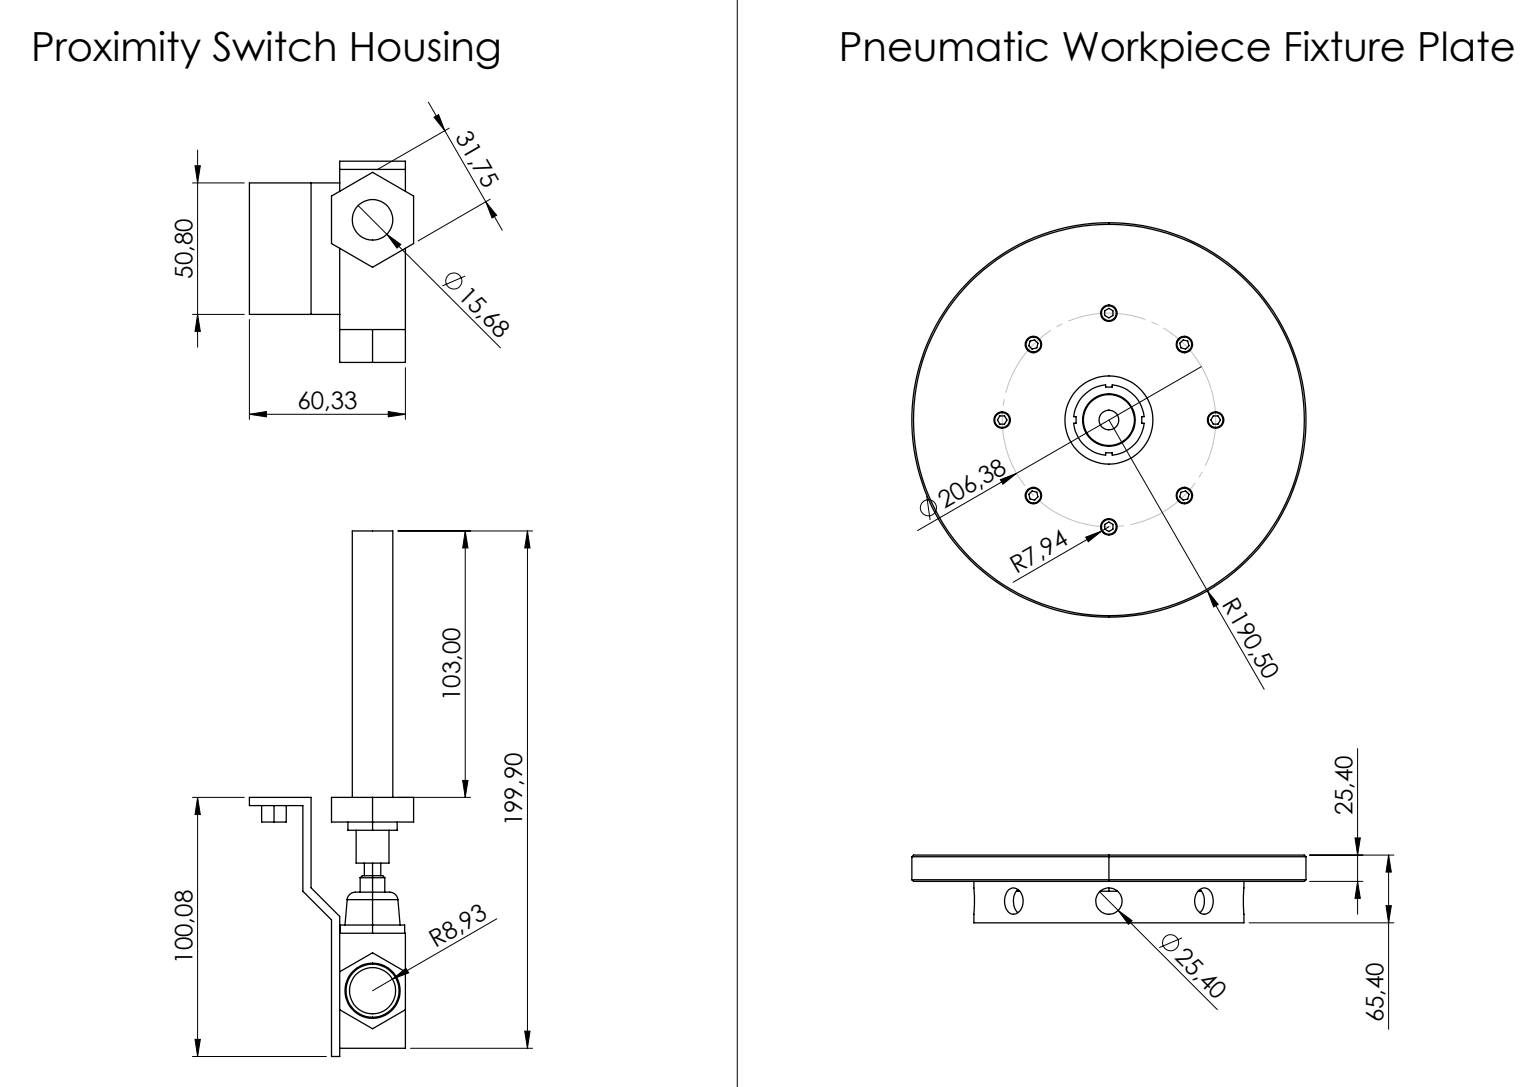
ISO-10303-21;
HEADER;
FILE_DESCRIPTION (('STEP AP214'),
    '1' );
FILE_NAME ('Proximity Switch Housing.step',
    '2026-10-07T11:37:37',
    ( '' ),
    ( '' ),
    'SwSTEP 2.0',
    'SolidWorks 2020',
    '' );
FILE_SCHEMA (( 'AUTOMOTIVE_DESIGN' ));
ENDSEC;

DATA;
#12=AXIS2_PLACEMENT_3D ( 'NONE', #30544, #63723, #30982 ) ;
#15=EDGE_LOOP ( 'NONE', ( #73624, #35100, #2042, #65680 ) ) ;
#24=CARTESIAN_POINT ( 'NONE',  ( 199.3900000000000148, 46.38749999999999574, -50.79999999999999716 ) ) ;
#109=ORIENTED_EDGE ( 'NONE', *, *, #12463, .F. ) ;
#113=DIRECTION ( 'NONE',  ( -1.000000000000000000, 0.000000000000000000, 0.000000000000000000 ) ) ;
#254=EDGE_CURVE ( 'NONE', #38623, #81994, #26176, .T. ) ;
#275=AXIS2_PLACEMENT_3D ( 'NONE', #19482, #13126, #74898 ) ;
#303=EDGE_CURVE ( 'NONE', #54782, #72244, #41574, .T. ) ;
#324=CARTESIAN_POINT ( 'NONE',  ( 199.3900000000000148, 59.08750000000000568, -50.79999999999999716 ) ) ;
#330=VECTOR ( 'NONE', #57470, 1000.000000000000000 ) ;
#479=LINE ( 'NONE', #75450, #54659 ) ;
#499=AXIS2_PLACEMENT_3D ( 'NONE', #66233, #38984, #31726 ) ;
#526=LINE ( 'NONE', #77290, #28220 ) ;
#540=DIRECTION ( 'NONE',  ( -1.000000000000000000, 0.000000000000000000, 0.000000000000000000 ) ) ;
#574=ORIENTED_EDGE ( 'NONE', *, *, #33050, .F. ) ;
#662=VECTOR ( 'NONE', #54108, 1000.000000000000000 ) ;
#687=VECTOR ( 'NONE', #72878, 1000.000000000000000 ) ;
#739=EDGE_CURVE ( 'NONE', #86672, #54266, #21377, .T. ) ;
#780=DIRECTION ( 'NONE',  ( -1.000000000000000000, 0.000000000000000000, 0.000000000000000000 ) ) ;
#832=PLANE ( 'NONE',  #52859 ) ;
#845=ORIENTED_EDGE ( 'NONE', *, *, #49423, .F. ) ;
#869=ADVANCED_FACE ( 'NONE', ( #70025 ), #14620, .F. ) ;
#917=DIRECTION ( 'NONE',  ( -1.000000000000000000, 3.651563665954184899E-16, 0.000000000000000000 ) ) ;
#1006=EDGE_CURVE ( 'NONE', #6675, #59868, #43643, .T. ) ;
#1029=EDGE_CURVE ( 'NONE', #69678, #54710, #73477, .T. ) ;
#1074=AXIS2_PLACEMENT_3D ( 'NONE', #83789, #85142, #1565 ) ;
#1102=EDGE_LOOP ( 'NONE', ( #66047, #88508, #70924, #49259 ) ) ;
#1110=CYLINDRICAL_SURFACE ( 'NONE', #1074, 3.174999999999997158 ) ;
#1150=ORIENTED_EDGE ( 'NONE', *, *, #9525, .F. ) ;
#1247=CIRCLE ( 'NONE', #51976, 6.647542495715439870 ) ;
#1266=CIRCLE ( 'NONE', #37574, 4.762500000000002842 ) ;
#1356=FACE_BOUND ( 'NONE', #25770, .T. ) ;
#1386=EDGE_CURVE ( 'NONE', #86177, #20936, #44319, .T. ) ;
#1433=CARTESIAN_POINT ( 'NONE',  ( 270.8910000000000196, 40.03750000000000142, -2.032000000000000028 ) ) ;
#1445=CARTESIAN_POINT ( 'NONE',  ( 183.5150000000000148, 36.86249999999999716, -53.61543552338530105 ) ) ;
#1493=EDGE_CURVE ( 'NONE', #9584, #8177, #75540, .T. ) ;
#1565=DIRECTION ( 'NONE',  ( 0.000000000000000000, 0.000000000000000000, 1.000000000000000000 ) ) ;
#1642=AXIS2_PLACEMENT_3D ( 'NONE', #6574, #49231, #61972 ) ;
#1645=PLANE ( 'NONE',  #8923 ) ;
#1649=LINE ( 'NONE', #29349, #83719 ) ;
#1671=ORIENTED_EDGE ( 'NONE', *, *, #58217, .F. ) ;
#1703=ORIENTED_EDGE ( 'NONE', *, *, #9525, .T. ) ;
#1756=ORIENTED_EDGE ( 'NONE', *, *, #68896, .F. ) ;
#1859=EDGE_LOOP ( 'NONE', ( #80684, #22830, #9417, #17174 ) ) ;
#1868=CARTESIAN_POINT ( 'NONE',  ( 219.9639999999999986, 40.03750000000000142, -58.73749999999999716 ) ) ;
#1873=VECTOR ( 'NONE', #29964, 1000.000000000000000 ) ;
#1909=LINE ( 'NONE', #56399, #17152 ) ;
#2007=DIRECTION ( 'NONE',  ( 1.000000000000000000, 0.000000000000000000, 0.000000000000000000 ) ) ;
#2029=ORIENTED_EDGE ( 'NONE', *, *, #65942, .T. ) ;
#2031=ORIENTED_EDGE ( 'NONE', *, *, #43091, .T. ) ;
#2042=ORIENTED_EDGE ( 'NONE', *, *, #74462, .F. ) ;
#2067=DIRECTION ( 'NONE',  ( 1.000000000000000000, 0.000000000000000000, 0.000000000000000000 ) ) ;
#2111=DIRECTION ( 'NONE',  ( -1.000000000000000000, 0.000000000000000000, -2.108231265501709878E-16 ) ) ;
#2112=AXIS2_PLACEMENT_3D ( 'NONE', #54801, #19863, #47549 ) ;
#2145=STYLED_ITEM ( 'NONE', ( #66142 ), #80104 ) ;
#2148=VECTOR ( 'NONE', #84868, 1000.000000000000000 ) ;
#2157=DIRECTION ( 'NONE',  ( -7.136255983449500255E-16, 0.000000000000000000, -1.000000000000000000 ) ) ;
#2234=ADVANCED_FACE ( 'NONE', ( #77753 ), #41852, .T. ) ;
#2261=LINE ( 'NONE', #50383, #1873 ) ;
#2282=CARTESIAN_POINT ( 'NONE',  ( 177.1649999999999920, 5.112500000000000711, -58.73749999999999716 ) ) ;
#2363=VECTOR ( 'NONE', #69256, 1000.000000000000000 ) ;
#2380=VECTOR ( 'NONE', #46487, 1000.000000000000000 ) ;
#2407=CARTESIAN_POINT ( 'NONE',  ( 270.8910000000000196, 40.03750000000000142, -67.11950000000000216 ) ) ;
#2427=AXIS2_PLACEMENT_3D ( 'NONE', #81072, #79730, #72455 ) ;
#2428=AXIS2_PLACEMENT_3D ( 'NONE', #75182, #5245, #32934 ) ;
#2439=DIRECTION ( 'NONE',  ( 1.000000000000000000, 0.000000000000000000, 0.000000000000000000 ) ) ;
#2482=CARTESIAN_POINT ( 'NONE',  ( 204.2160000000000082, 52.73749999999999716, -40.48124999999945572 ) ) ;
#2499=EDGE_CURVE ( 'NONE', #28622, #16389, #84475, .T. ) ;
#2686=DIRECTION ( 'NONE',  ( 0.000000000000000000, 0.000000000000000000, 1.000000000000000000 ) ) ;
#2696=LINE ( 'NONE', #16767, #70704 ) ;
#2727=VERTEX_POINT ( 'NONE', #73946 ) ;
#2742=DIRECTION ( 'NONE',  ( 0.000000000000000000, 0.000000000000000000, -1.000000000000000000 ) ) ;
#2848=CARTESIAN_POINT ( 'NONE',  ( 226.4410000000000025, 40.03750000000000142, 10.66800000000000104 ) ) ;
#2953=VERTEX_POINT ( 'NONE', #86482 ) ;
#2982=VERTEX_POINT ( 'NONE', #59630 ) ;
#2985=VERTEX_POINT ( 'NONE', #38308 ) ;
#3007=AXIS2_PLACEMENT_3D ( 'NONE', #78593, #71762, #83602 ) ;
#3067=DIRECTION ( 'NONE',  ( -1.000000000000000000, 0.000000000000000000, -2.108231265501709878E-16 ) ) ;
#3078=VECTOR ( 'NONE', #53283, 1000.000000000000000 ) ;
#3128=ORIENTED_EDGE ( 'NONE', *, *, #41850, .T. ) ;
#3145=DIRECTION ( 'NONE',  ( 0.000000000000000000, -0.8660254037844383745, -0.5000000000000003331 ) ) ;
#3249=VECTOR ( 'NONE', #48898, 1000.000000000000000 ) ;
#3299=SURFACE_STYLE_USAGE ( .BOTH. , #17812 ) ;
#3320=ORIENTED_EDGE ( 'NONE', *, *, #23264, .T. ) ;
#3451=CARTESIAN_POINT ( 'NONE',  ( 223.2659999999999911, 52.73749999999999716, -32.00399999999999778 ) ) ;
#3471=EDGE_CURVE ( 'NONE', #54390, #10350, #12838, .T. ) ;
#3643=CARTESIAN_POINT ( 'NONE',  ( 177.1649999999999920, 5.112500000000000711, -7.937500000000000000 ) ) ;
#3651=CIRCLE ( 'NONE', #41367, 10.26166025953212468 ) ;
#3667=CARTESIAN_POINT ( 'NONE',  ( 223.2659999999999911, 52.73749999999999716, -44.45000000000000284 ) ) ;
#3711=DIRECTION ( 'NONE',  ( 1.000000000000000000, 0.000000000000000000, 0.000000000000000000 ) ) ;
#3736=( LENGTH_UNIT ( ) NAMED_UNIT ( * ) SI_UNIT ( .MILLI., .METRE. ) );
#3760=ORIENTED_EDGE ( 'NONE', *, *, #23279, .T. ) ;
#3831=VERTEX_POINT ( 'NONE', #85830 ) ;
#3838=VECTOR ( 'NONE', #48336, 1000.000000000000000 ) ;
#3867=CARTESIAN_POINT ( 'NONE',  ( 173.9899999999999807, 52.73749999999999716, -52.28750000000000142 ) ) ;
#3937=ORIENTED_EDGE ( 'NONE', *, *, #41802, .T. ) ;
#4117=CARTESIAN_POINT ( 'NONE',  ( 173.9900000000000091, 52.73749999999999716, -62.78087104677060637 ) ) ;
#4160=CARTESIAN_POINT ( 'NONE',  ( 223.2659999999999911, 52.73749999999999716, -32.00399999999999778 ) ) ;
#4201=CARTESIAN_POINT ( 'NONE',  ( 177.1649999999999920, 14.63749999999999929, -52.38749999999999574 ) ) ;
#4243=DIRECTION ( 'NONE',  ( 1.000000000000000000, -0.000000000000000000, 2.108231265501710124E-16 ) ) ;
#4288=CARTESIAN_POINT ( 'NONE',  ( 183.5150000000000148, 52.73749999999999716, -26.11912895322935313 ) ) ;
#4323=ORIENTED_EDGE ( 'NONE', *, *, #74462, .T. ) ;
#4489=EDGE_CURVE ( 'NONE', #56634, #71751, #79798, .T. ) ;
#4515=ORIENTED_EDGE ( 'NONE', *, *, #27620, .F. ) ;
#4572=VECTOR ( 'NONE', #22994, 1000.000000000000000 ) ;
#4580=EDGE_LOOP ( 'NONE', ( #33206, #53501, #39020, #4323, #51486, #11776 ) ) ;
#4611=VERTEX_POINT ( 'NONE', #71043 ) ;
#4729=PLANE ( 'NONE',  #67107 ) ;
#4776=EDGE_CURVE ( 'NONE', #88384, #78380, #88690, .T. ) ;
#4790=EDGE_CURVE ( 'NONE', #2982, #52784, #78320, .T. ) ;
#4815=DIRECTION ( 'NONE',  ( -1.000000000000000000, 0.000000000000000000, 0.000000000000000000 ) ) ;
#4819=ORIENTED_EDGE ( 'NONE', *, *, #87208, .F. ) ;
#4821=CIRCLE ( 'NONE', #38214, 4.762500000000002842 ) ;
#4869=VECTOR ( 'NONE', #26634, 1000.000000000000000 ) ;
#4881=DIRECTION ( 'NONE',  ( 0.000000000000000000, 0.000000000000000000, 1.000000000000000000 ) ) ;
#4896=DIRECTION ( 'NONE',  ( -7.980413499659419871E-32, 1.000000000000000000, 3.785359618865284342E-16 ) ) ;
#4921=FACE_OUTER_BOUND ( 'NONE', #41166, .T. ) ;
#4941=EDGE_CURVE ( 'NONE', #64462, #86177, #25609, .T. ) ;
#4972=LINE ( 'NONE', #60365, #32186 ) ;
#5049=LINE ( 'NONE', #45024, #11322 ) ;
#5066=ORIENTED_EDGE ( 'NONE', *, *, #16121, .T. ) ;
#5245=DIRECTION ( 'NONE',  ( 0.000000000000000000, -1.000000000000000000, 0.000000000000000000 ) ) ;
#5445=LINE ( 'NONE', #68114, #10349 ) ;
#5493=DIRECTION ( 'NONE',  ( 0.000000000000000000, 0.000000000000000000, 1.000000000000000000 ) ) ;
#5642=DIRECTION ( 'NONE',  ( 1.000000000000000000, 0.000000000000000000, 0.000000000000000000 ) ) ;
#5664=EDGE_CURVE ( 'NONE', #22107, #30158, #47504, .T. ) ;
#5881=CARTESIAN_POINT ( 'NONE',  ( 173.9900000000000091, 5.112500000000000711, -7.937500000000000000 ) ) ;
#5942=CARTESIAN_POINT ( 'NONE',  ( 223.2659999999999911, 36.86249999999999716, -2.032000000000000028 ) ) ;
#6110=DIRECTION ( 'NONE',  ( -1.000000000000000000, 0.000000000000000000, 0.000000000000000000 ) ) ;
#6112=DIRECTION ( 'NONE',  ( -1.000000000000000000, 0.000000000000000000, 0.000000000000000000 ) ) ;
#6116=ORIENTED_EDGE ( 'NONE', *, *, #76740, .T. ) ;
#6360=VERTEX_POINT ( 'NONE', #29660 ) ;
#6379=EDGE_LOOP ( 'NONE', ( #29242, #79517, #85233, #49817, #49646, #1703 ) ) ;
#6410=EDGE_CURVE ( 'NONE', #78558, #73485, #7548, .T. ) ;
#6437=VECTOR ( 'NONE', #780, 1000.000000000000000 ) ;
#6476=AXIS2_PLACEMENT_3D ( 'NONE', #8190, #42680, #69522 ) ;
#6480=CIRCLE ( 'NONE', #74626, 12.44599999999999795 ) ;
#6490=DIRECTION ( 'NONE',  ( -0.8660254037844387076, 0.4999999999999998890, 0.000000000000000000 ) ) ;
#6491=EDGE_CURVE ( 'NONE', #47477, #14995, #80961, .T. ) ;
#6512=DIRECTION ( 'NONE',  ( 0.000000000000000000, 0.000000000000000000, -1.000000000000000000 ) ) ;
#6526=CIRCLE ( 'NONE', #45655, 3.174999999999997158 ) ;
#6546=LINE ( 'NONE', #81085, #16069 ) ;
#6574=CARTESIAN_POINT ( 'NONE',  ( 183.5150000000000148, 14.63749999999999929, -14.28749999999999964 ) ) ;
#6654=DIRECTION ( 'NONE',  ( 0.7071067811865504593, 0.000000000000000000, 0.7071067811865445751 ) ) ;
#6662=VECTOR ( 'NONE', #57712, 1000.000000000000000 ) ;
#6671=DIRECTION ( 'NONE',  ( 0.000000000000000000, 0.000000000000000000, -1.000000000000000000 ) ) ;
#6675=VERTEX_POINT ( 'NONE', #55889 ) ;
#6744=CARTESIAN_POINT ( 'NONE',  ( 183.5150000000000148, 68.61249999999999716, -35.28456447661459805 ) ) ;
#6795=EDGE_CURVE ( 'NONE', #65795, #61431, #32119, .T. ) ;
#6839=VECTOR ( 'NONE', #25383, 1000.000000000000000 ) ;
#6841=ORIENTED_EDGE ( 'NONE', *, *, #55333, .F. ) ;
#6894=LINE ( 'NONE', #22330, #26794 ) ;
#7063=ORIENTED_EDGE ( 'NONE', *, *, #81554, .T. ) ;
#7112=DIRECTION ( 'NONE',  ( 0.000000000000000000, 0.000000000000000000, 1.000000000000000000 ) ) ;
#7131=EDGE_CURVE ( 'NONE', #15176, #54672, #85227, .T. ) ;
#7165=( GEOMETRIC_REPRESENTATION_CONTEXT ( 3 ) GLOBAL_UNCERTAINTY_ASSIGNED_CONTEXT ( ( #28762 ) ) GLOBAL_UNIT_ASSIGNED_CONTEXT ( ( #3736, #71897, #44158 ) ) REPRESENTATION_CONTEXT ( 'NONE', 'WORKASPACE' ) );
#7203=ORIENTED_EDGE ( 'NONE', *, *, #5664, .F. ) ;
#7223=ORIENTED_EDGE ( 'NONE', *, *, #30920, .T. ) ;
#7285=ORIENTED_EDGE ( 'NONE', *, *, #44170, .T. ) ;
#7290=FACE_OUTER_BOUND ( 'NONE', #87103, .T. ) ;
#7453=ORIENTED_EDGE ( 'NONE', *, *, #30720, .T. ) ;
#7485=EDGE_CURVE ( 'NONE', #81994, #84665, #6546, .T. ) ;
#7493=LINE ( 'NONE', #35178, #50384 ) ;
#7548=CIRCLE ( 'NONE', #19148, 9.810460662156732070 ) ;
#7583=CARTESIAN_POINT ( 'NONE',  ( 204.2160000000000082, 52.73749999999999716, -40.48124999999945572 ) ) ;
#7617=ORIENTED_EDGE ( 'NONE', *, *, #1493, .F. ) ;
#7626=DIRECTION ( 'NONE',  ( 0.000000000000000000, 0.000000000000000000, 1.000000000000000000 ) ) ;
#7653=CARTESIAN_POINT ( 'NONE',  ( 270.8910000000000196, 65.43750000000000000, -2.032000000000000028 ) ) ;
#7681=PLANE ( 'NONE',  #27434 ) ;
#7809=FACE_OUTER_BOUND ( 'NONE', #85300, .T. ) ;
#7840=DIRECTION ( 'NONE',  ( 0.000000000000000000, 0.000000000000000000, -1.000000000000000000 ) ) ;
#7843=DIRECTION ( 'NONE',  ( 0.000000000000000000, 0.000000000000000000, 1.000000000000000000 ) ) ;
#7994=PLANE ( 'NONE',  #50960 ) ;
#8009=AXIS2_PLACEMENT_3D ( 'NONE', #64340, #2111, #29821 ) ;
#8064=EDGE_LOOP ( 'NONE', ( #83886, #3320, #1150, #32681, #73638, #52637, #41775, #28996 ) ) ;
#8075=DIRECTION ( 'NONE',  ( -1.000000000000000000, 0.000000000000000000, -2.108231265501709878E-16 ) ) ;
#8113=ORIENTED_EDGE ( 'NONE', *, *, #80354, .F. ) ;
#8158=EDGE_LOOP ( 'NONE', ( #20110, #78432, #2029, #49660 ) ) ;
#8177=VERTEX_POINT ( 'NONE', #79977 ) ;
#8190=CARTESIAN_POINT ( 'NONE',  ( 183.5150000000000148, 14.63749999999999929, -52.38749999999999574 ) ) ;
#8302=FACE_BOUND ( 'NONE', #23000, .T. ) ;
#8349=EDGE_CURVE ( 'NONE', #47225, #2985, #5445, .T. ) ;
#8374=ADVANCED_FACE ( 'NONE', ( #46298, #31794, #12251 ), #39944, .F. ) ;
#8429=ORIENTED_EDGE ( 'NONE', *, *, #4489, .F. ) ;
#8455=CARTESIAN_POINT ( 'NONE',  ( 248.6659999999999968, 52.73749999999999716, 10.66800000000000104 ) ) ;
#8461=ORIENTED_EDGE ( 'NONE', *, *, #57159, .T. ) ;
#8474=DIRECTION ( 'NONE',  ( -1.000000000000000000, 0.000000000000000000, 5.463695987328529395E-16 ) ) ;
#8565=VERTEX_POINT ( 'NONE', #56243 ) ;
#8726=CARTESIAN_POINT ( 'NONE',  ( 270.8910000000000196, 40.03750000000000142, -7.937500000000000000 ) ) ;
#8761=PLANE ( 'NONE',  #54111 ) ;
#8850=DIRECTION ( 'NONE',  ( 0.000000000000000000, 0.000000000000000000, 1.000000000000000000 ) ) ;
#8864=CARTESIAN_POINT ( 'NONE',  ( 205.0097499999990305, 52.73749999999999716, -49.21249999999999858 ) ) ;
#8923=AXIS2_PLACEMENT_3D ( 'NONE', #50209, #28430, #36611 ) ;
#8938=ORIENTED_EDGE ( 'NONE', *, *, #10937, .F. ) ;
#9003=ORIENTED_EDGE ( 'NONE', *, *, #13599, .F. ) ;
#9037=VERTEX_POINT ( 'NONE', #60159 ) ;
#9061=ORIENTED_EDGE ( 'NONE', *, *, #13025, .T. ) ;
#9154=VECTOR ( 'NONE', #28074, 1000.000000000000000 ) ;
#9187=CARTESIAN_POINT ( 'NONE',  ( 183.5150000000000148, 14.63749999999999929, -9.525000000000000355 ) ) ;
#9237=CARTESIAN_POINT ( 'NONE',  ( 263.3306968374159851, 52.73749999999999716, -2.032000000000000028 ) ) ;
#9264=CARTESIAN_POINT ( 'NONE',  ( 205.0097499999990305, 52.73749999999999716, -44.45000000000000284 ) ) ;
#9417=ORIENTED_EDGE ( 'NONE', *, *, #83533, .T. ) ;
#9525=EDGE_CURVE ( 'NONE', #62756, #15555, #526, .T. ) ;
#9570=DIRECTION ( 'NONE',  ( -1.000000000000000000, 0.000000000000000000, -2.108231265501709878E-16 ) ) ;
#9577=LINE ( 'NONE', #87220, #70374 ) ;
#9584=VERTEX_POINT ( 'NONE', #55916 ) ;
#9589=EDGE_CURVE ( 'NONE', #84035, #35999, #6894, .T. ) ;
#9637=ORIENTED_EDGE ( 'NONE', *, *, #10817, .T. ) ;
#9639=DIRECTION ( 'NONE',  ( 0.000000000000000000, -1.000000000000000000, 0.000000000000000000 ) ) ;
#9649=LINE ( 'NONE', #2848, #27057 ) ;
#9678=VECTOR ( 'NONE', #2686, 1000.000000000000000 ) ;
#9707=DIRECTION ( 'NONE',  ( 1.000000000000000000, 0.000000000000000000, 0.000000000000000000 ) ) ;
#9795=CIRCLE ( 'NONE', #75074, 12.44599999999999795 ) ;
#9866=ORIENTED_EDGE ( 'NONE', *, *, #41587, .F. ) ;
#9890=CARTESIAN_POINT ( 'NONE',  ( 257.5940999999999690, 52.73749999999999716, 10.66800000000000104 ) ) ;
#9978=DIRECTION ( 'NONE',  ( 0.000000000000000000, 0.000000000000000000, 1.000000000000000000 ) ) ;
#9984=CARTESIAN_POINT ( 'NONE',  ( 183.5150000000000148, 68.61249999999999716, -53.61543552338530105 ) ) ;
#10068=AXIS2_PLACEMENT_3D ( 'NONE', #58861, #24807, #66576 ) ;
#10192=ORIENTED_EDGE ( 'NONE', *, *, #9589, .F. ) ;
#10279=ORIENTED_EDGE ( 'NONE', *, *, #62430, .T. ) ;
#10290=ORIENTED_EDGE ( 'NONE', *, *, #57784, .T. ) ;
#10349=VECTOR ( 'NONE', #13155, 1000.000000000000000 ) ;
#10350=VERTEX_POINT ( 'NONE', #3451 ) ;
#10356=DIRECTION ( 'NONE',  ( 2.108231265501709878E-16, 0.000000000000000000, -1.000000000000000000 ) ) ;
#10368=DIRECTION ( 'NONE',  ( 0.000000000000000000, 0.000000000000000000, 1.000000000000000000 ) ) ;
#10440=DIRECTION ( 'NONE',  ( 0.000000000000000000, 0.000000000000000000, 1.000000000000000000 ) ) ;
#10536=CIRCLE ( 'NONE', #22159, 4.762500000000002842 ) ;
#10560=CARTESIAN_POINT ( 'NONE',  ( 186.6899999999999977, 59.08750000000000568, -50.79999999999999716 ) ) ;
#10635=ADVANCED_FACE ( 'NONE', ( #78327 ), #1110, .T. ) ;
#10645=CARTESIAN_POINT ( 'NONE',  ( 204.2160000000000082, 52.73749999999999716, -44.45000000000000284 ) ) ;
#10666=DIRECTION ( 'NONE',  ( 0.000000000000000000, 1.000000000000000000, 5.463695987328529395E-16 ) ) ;
#10732=( NAMED_UNIT ( * ) PLANE_ANGLE_UNIT ( ) SI_UNIT ( $, .RADIAN. ) );
#10739=LINE ( 'NONE', #23516, #49588 ) ;
#10781=AXIS2_PLACEMENT_3D ( 'NONE', #85648, #66056, #17039 ) ;
#10817=EDGE_CURVE ( 'NONE', #2727, #42703, #82392, .T. ) ;
#10845=VERTEX_POINT ( 'NONE', #82343 ) ;
#10919=EDGE_CURVE ( 'NONE', #32855, #84272, #82794, .T. ) ;
#10937=EDGE_CURVE ( 'NONE', #25134, #76956, #36857, .T. ) ;
#10944=DIRECTION ( 'NONE',  ( 1.000000000000000000, 0.000000000000000000, -5.463695987328529395E-16 ) ) ;
#10984=CIRCLE ( 'NONE', #21120, 9.524999999999998579 ) ;
#10990=( NAMED_UNIT ( * ) PLANE_ANGLE_UNIT ( ) SI_UNIT ( $, .RADIAN. ) );
#11060=FACE_OUTER_BOUND ( 'NONE', #54415, .T. ) ;
#11080=DIRECTION ( 'NONE',  ( 0.9961946980917455452, 0.000000000000000000, 0.08715574274765836016 ) ) ;
#11094=DIRECTION ( 'NONE',  ( 0.000000000000000000, 0.000000000000000000, 1.000000000000000000 ) ) ;
#11154=CARTESIAN_POINT ( 'NONE',  ( 241.3336515812914911, 65.43750000000000000, -2.032000000000000028 ) ) ;
#11195=VERTEX_POINT ( 'NONE', #4117 ) ;
#11229=VECTOR ( 'NONE', #22249, 1000.000000000000000 ) ;
#11246=ORIENTED_EDGE ( 'NONE', *, *, #42075, .F. ) ;
#11253=PLANE ( 'NONE',  #83559 ) ;
#11306=VECTOR ( 'NONE', #80656, 1000.000000000000000 ) ;
#11322=VECTOR ( 'NONE', #18675, 1000.000000000000000 ) ;
#11404=ORIENTED_EDGE ( 'NONE', *, *, #32887, .F. ) ;
#11437=EDGE_CURVE ( 'NONE', #30447, #18949, #70377, .T. ) ;
#11451=DIRECTION ( 'NONE',  ( -1.825781832977099352E-16, 0.4999999999999998890, 0.8660254037844387076 ) ) ;
#11465=CARTESIAN_POINT ( 'NONE',  ( 199.3900000000000148, 52.73749999999999716, -44.45000000000000284 ) ) ;
#11513=LINE ( 'NONE', #39209, #44408 ) ;
#11535=EDGE_CURVE ( 'NONE', #74351, #54417, #57629, .T. ) ;
#11587=AXIS2_PLACEMENT_3D ( 'NONE', #32865, #46926, #31972 ) ;
#11687=DIRECTION ( 'NONE',  ( -2.108231265501709878E-16, 5.463695987328529395E-16, 1.000000000000000000 ) ) ;
#11776=ORIENTED_EDGE ( 'NONE', *, *, #45978, .T. ) ;
#11779=ORIENTED_EDGE ( 'NONE', *, *, #64075, .T. ) ;
#11829=ADVANCED_FACE ( 'NONE', ( #40311 ), #27257, .T. ) ;
#11853=AXIS2_PLACEMENT_3D ( 'NONE', #81263, #79476, #31288 ) ;
#11871=CARTESIAN_POINT ( 'NONE',  ( 204.2160000000000082, 52.73749999999999716, -48.41875000000000284 ) ) ;
#11875=AXIS2_PLACEMENT_3D ( 'NONE', #17373, #86429, #45056 ) ;
#11891=EDGE_CURVE ( 'NONE', #52784, #11922, #48008, .T. ) ;
#11894=FACE_OUTER_BOUND ( 'NONE', #30527, .T. ) ;
#11922=VERTEX_POINT ( 'NONE', #41200 ) ;
#11931=CARTESIAN_POINT ( 'NONE',  ( 173.9900000000000091, 52.73749999999999716, -26.11912895322935313 ) ) ;
#11948=DIRECTION ( 'NONE',  ( 1.000000000000000000, 1.314511288311335947E-16, 0.000000000000000000 ) ) ;
#11981=ORIENTED_EDGE ( 'NONE', *, *, #17799, .T. ) ;
#12025=DIRECTION ( 'NONE',  ( 0.000000000000000000, 0.000000000000000000, -1.000000000000000000 ) ) ;
#12026=CARTESIAN_POINT ( 'NONE',  ( 183.5150000000000148, 14.63749999999999929, -52.38749999999999574 ) ) ;
#12175=EDGE_CURVE ( 'NONE', #83823, #14890, #27368, .T. ) ;
#12249=LINE ( 'NONE', #61282, #13166 ) ;
#12251=FACE_BOUND ( 'NONE', #56681, .T. ) ;
#12273=DIRECTION ( 'NONE',  ( 0.000000000000000000, -0.8660254037844383745, -0.5000000000000003331 ) ) ;
#12325=EDGE_CURVE ( 'NONE', #83557, #61431, #35513, .T. ) ;
#12329=PLANE ( 'NONE',  #33594 ) ;
#12369=CARTESIAN_POINT ( 'NONE',  ( 183.5150000000000148, 52.73749999999999716, -34.92499999999999716 ) ) ;
#12402=VECTOR ( 'NONE', #59601, 1000.000000000000000 ) ;
#12416=CARTESIAN_POINT ( 'NONE',  ( 204.2160000000000082, 52.73749999999999716, -48.41875000000000284 ) ) ;
#12435=CARTESIAN_POINT ( 'NONE',  ( 183.5150000000000148, 68.61249999999999716, -71.94630657015589748 ) ) ;
#12459=ADVANCED_FACE ( 'NONE', ( #85939 ), #87702, .F. ) ;
#12463=EDGE_CURVE ( 'NONE', #17992, #69275, #53138, .T. ) ;
#12464=CARTESIAN_POINT ( 'NONE',  ( 204.2160000000000082, 52.73749999999999716, -39.68750000000000000 ) ) ;
#12470=FACE_OUTER_BOUND ( 'NONE', #60850, .T. ) ;
#12473=EDGE_CURVE ( 'NONE', #66028, #64424, #52875, .T. ) ;
#12496=ORIENTED_EDGE ( 'NONE', *, *, #68896, .T. ) ;
#12522=EDGE_LOOP ( 'NONE', ( #37000, #71430, #23849, #81883 ) ) ;
#12595=ADVANCED_FACE ( 'NONE', ( #40440 ), #68609, .T. ) ;
#12709=DIRECTION ( 'NONE',  ( -1.000000000000000000, 0.000000000000000000, 0.000000000000000000 ) ) ;
#12759=VERTEX_POINT ( 'NONE', #47540 ) ;
#12838=CIRCLE ( 'NONE', #56310, 12.44599999999999795 ) ;
#12839=VERTEX_POINT ( 'NONE', #70244 ) ;
#12943=FACE_BOUND ( 'NONE', #47307, .T. ) ;
#13000=EDGE_CURVE ( 'NONE', #9037, #88384, #15292, .T. ) ;
#13006=CARTESIAN_POINT ( 'NONE',  ( 208.9149999999999920, 28.98850000000000193, -58.73749999999999716 ) ) ;
#13025=EDGE_CURVE ( 'NONE', #54266, #86672, #3651, .T. ) ;
#13087=PLANE ( 'NONE',  #39711 ) ;
#13126=DIRECTION ( 'NONE',  ( 1.000000000000000000, -0.000000000000000000, 2.108231265501710124E-16 ) ) ;
#13142=EDGE_LOOP ( 'NONE', ( #76348, #845, #5066, #62903 ) ) ;
#13155=DIRECTION ( 'NONE',  ( -1.000000000000000000, 0.000000000000000000, -2.108231265501709878E-16 ) ) ;
#13166=VECTOR ( 'NONE', #39942, 1000.000000000000114 ) ;
#13179=AXIS2_PLACEMENT_3D ( 'NONE', #13990, #8075, #7626 ) ;
#13209=CARTESIAN_POINT ( 'NONE',  ( 242.3160000000000025, 65.43750000000000000, -63.94449999999999790 ) ) ;
#13223=VERTEX_POINT ( 'NONE', #11931 ) ;
#13285=ADVANCED_FACE ( 'NONE', ( #80530 ), #45521, .F. ) ;
#13321=ORIENTED_EDGE ( 'NONE', *, *, #49065, .F. ) ;
#13322=LINE ( 'NONE', #62353, #32835 ) ;
#13353=DIRECTION ( 'NONE',  ( 0.4999999999999998890, -0.8660254037844387076, 0.000000000000000000 ) ) ;
#13416=EDGE_LOOP ( 'NONE', ( #1671, #34448, #3937, #43491 ) ) ;
#13430=DIRECTION ( 'NONE',  ( 1.000000000000000000, 0.000000000000000000, 0.000000000000000000 ) ) ;
#13492=ORIENTED_EDGE ( 'NONE', *, *, #31313, .F. ) ;
#13566=VERTEX_POINT ( 'NONE', #1445 ) ;
#13599=EDGE_CURVE ( 'NONE', #24899, #81994, #72714, .T. ) ;
#13682=ADVANCED_FACE ( 'NONE', ( #80424 ), #66776, .T. ) ;
#13802=ADVANCED_FACE ( 'NONE', ( #26344 ), #54013, .F. ) ;
#13830=ORIENTED_EDGE ( 'NONE', *, *, #58217, .T. ) ;
#13905=LINE ( 'NONE', #29336, #330 ) ;
#13920=PLANE ( 'NONE',  #60482 ) ;
#13990=CARTESIAN_POINT ( 'NONE',  ( 173.9899999999999807, 52.73749999999999716, -44.45000000000000284 ) ) ;
#14024=LINE ( 'NONE', #5881, #16272 ) ;
#14146=PLANE ( 'NONE',  #42882 ) ;
#14163=DIRECTION ( 'NONE',  ( -1.000000000000000000, 0.000000000000000000, -2.108231265501709878E-16 ) ) ;
#14191=DIRECTION ( 'NONE',  ( 0.000000000000000000, 0.000000000000000000, 1.000000000000000000 ) ) ;
#14206=EDGE_CURVE ( 'NONE', #40315, #14995, #55588, .T. ) ;
#14228=FACE_OUTER_BOUND ( 'NONE', #85742, .T. ) ;
#14268=VECTOR ( 'NONE', #19301, 1000.000000000000000 ) ;
#14283=FACE_OUTER_BOUND ( 'NONE', #77955, .T. ) ;
#14323=DIRECTION ( 'NONE',  ( 1.000000000000000000, 0.000000000000000000, 0.000000000000000000 ) ) ;
#14335=ORIENTED_EDGE ( 'NONE', *, *, #30920, .F. ) ;
#14351=DIRECTION ( 'NONE',  ( -0.4999999999999998890, -0.8660254037844387076, 0.000000000000000000 ) ) ;
#14364=APPLICATION_CONTEXT ( 'automotive_design' ) ;
#14478=ORIENTED_EDGE ( 'NONE', *, *, #72954, .F. ) ;
#14504=ORIENTED_EDGE ( 'NONE', *, *, #16889, .F. ) ;
#14507=FACE_BOUND ( 'NONE', #88844, .T. ) ;
#14568=AXIS2_PLACEMENT_3D ( 'NONE', #75660, #13430, #24080 ) ;
#14571=ORIENTED_EDGE ( 'NONE', *, *, #19847, .F. ) ;
#14590=CONICAL_SURFACE ( 'NONE', #49373, 10.66799999999999748, 0.08726646259971625186 ) ;
#14620=PLANE ( 'NONE',  #85268 ) ;
#14802=ORIENTED_EDGE ( 'NONE', *, *, #4790, .T. ) ;
#14874=VECTOR ( 'NONE', #11080, 1000.000000000000114 ) ;
#14890=VERTEX_POINT ( 'NONE', #8726 ) ;
#14922=DIRECTION ( 'NONE',  ( 1.000000000000000000, 0.000000000000000000, 2.108231265501709878E-16 ) ) ;
#14938=EDGE_LOOP ( 'NONE', ( #57231, #35001, #27329, #12496 ) ) ;
#14971=CARTESIAN_POINT ( 'NONE',  ( 255.9983484187079910, 40.03750000000000142, -2.032000000000000028 ) ) ;
#14995=VERTEX_POINT ( 'NONE', #81351 ) ;
#15066=CARTESIAN_POINT ( 'NONE',  ( 226.4410000000000025, 52.73749999999999716, -56.89600000000000080 ) ) ;
#15087=DIRECTION ( 'NONE',  ( 1.000000000000000000, 0.000000000000000000, 3.902639990948949304E-17 ) ) ;
#15176=VERTEX_POINT ( 'NONE', #28585 ) ;
#15191=ORIENTED_EDGE ( 'NONE', *, *, #30986, .T. ) ;
#15292=LINE ( 'NONE', #42961, #48617 ) ;
#15302=DIRECTION ( 'NONE',  ( 0.000000000000000000, 0.000000000000000000, 1.000000000000000000 ) ) ;
#15371=CARTESIAN_POINT ( 'NONE',  ( 274.0659999999999741, 40.03750000000000142, -7.937500000000000000 ) ) ;
#15385=CARTESIAN_POINT ( 'NONE',  ( 183.5150000000000148, 52.73749999999999716, -53.97500000000000142 ) ) ;
#15406=VECTOR ( 'NONE', #12273, 1000.000000000000114 ) ;
#15472=LINE ( 'NONE', #2282, #64343 ) ;
#15548=DIRECTION ( 'NONE',  ( 1.000000000000000000, -0.000000000000000000, 2.108231265501710124E-16 ) ) ;
#15549=CLOSED_SHELL ( 'NONE', ( #74468, #26821, #67375, #13285, #28353, #65151, #33795, #77184, #84683, #31319, #24361, #16466, #24022, #52408, #17074, #83080, #48006, #23673, #10635, #83086, #25602, #76205, #35146, #77355, #26934, #26632, #869, #34880, #8374, #85557, #82623, #34634, #56960, #17157, #49843, #28210, #2234, #55795, #57273, #26920, #79966, #49808, #74242, #12595, #63022, #84677, #74077, #32482, #54691, #52567, #12459, #30017, #66107, #13802, #21394, #13682, #16914, #38862, #73046, #31934, #60432, #16702, #81389, #44852, #52770, #28853, #35826, #11829, #34859, #80259, #48452, #23756, #75841, #33007 ) ) ;
#15555=VERTEX_POINT ( 'NONE', #29844 ) ;
#15586=CARTESIAN_POINT ( 'NONE',  ( 70.98999999999998067, 52.73749999999999716, -52.28750000000002274 ) ) ;
#15633=ORIENTED_EDGE ( 'NONE', *, *, #50626, .F. ) ;
#15705=CYLINDRICAL_SURFACE ( 'NONE', #57204, 4.762500000000001066 ) ;
#15816=LINE ( 'NONE', #9890, #2148 ) ;
#15916=FACE_OUTER_BOUND ( 'NONE', #86387, .T. ) ;
#16012=VECTOR ( 'NONE', #80001, 1000.000000000000000 ) ;
#16015=DIRECTION ( 'NONE',  ( 1.000000000000000000, 0.000000000000000000, 0.000000000000000000 ) ) ;
#16040=PRESENTATION_STYLE_ASSIGNMENT (( #3299 ) ) ;
#16069=VECTOR ( 'NONE', #6112, 1000.000000000000000 ) ;
#16111=VECTOR ( 'NONE', #82501, 999.9999999999998863 ) ;
#16121=EDGE_CURVE ( 'NONE', #60085, #4611, #57764, .T. ) ;
#16130=VECTOR ( 'NONE', #18782, 1000.000000000000000 ) ;
#16152=CARTESIAN_POINT ( 'NONE',  ( 226.4410000000000025, 40.03750000000000142, -2.032000000000000028 ) ) ;
#16200=CARTESIAN_POINT ( 'NONE',  ( 223.2659999999999911, 52.73749999999999716, -55.11800000000000210 ) ) ;
#16272=VECTOR ( 'NONE', #75363, 1000.000000000000000 ) ;
#16308=CARTESIAN_POINT ( 'NONE',  ( 177.1649999999999920, 25.81350000000000477, -58.73749999999999716 ) ) ;
#16343=DIRECTION ( 'NONE',  ( 0.000000000000000000, 0.000000000000000000, 1.000000000000000000 ) ) ;
#16361=VECTOR ( 'NONE', #79725, 1000.000000000000000 ) ;
#16373=EDGE_CURVE ( 'NONE', #30447, #6360, #89051, .T. ) ;
#16389=VERTEX_POINT ( 'NONE', #77222 ) ;
#16450=CARTESIAN_POINT ( 'NONE',  ( 183.5150000000000148, 36.86249999999999716, -53.61543552338530105 ) ) ;
#16466=ADVANCED_FACE ( 'NONE', ( #23173 ), #72192, .T. ) ;
#16493=FACE_OUTER_BOUND ( 'NONE', #14938, .T. ) ;
#16518=EDGE_CURVE ( 'NONE', #2985, #13223, #2261, .T. ) ;
#16539=LINE ( 'NONE', #44214, #68538 ) ;
#16552=DIRECTION ( 'NONE',  ( -2.108231265501709878E-16, 0.000000000000000000, 1.000000000000000000 ) ) ;
#16597=DIRECTION ( 'NONE',  ( 0.000000000000000000, 0.000000000000000000, 1.000000000000000000 ) ) ;
#16609=CYLINDRICAL_SURFACE ( 'NONE', #31261, 4.762500000000001066 ) ;
#16683=EDGE_LOOP ( 'NONE', ( #34049, #13492, #37190, #33205 ) ) ;
#16688=CARTESIAN_POINT ( 'NONE',  ( 258.9276602595319901, 52.73749999999999716, -2.903194600000015502 ) ) ;
#16702=ADVANCED_FACE ( 'NONE', ( #33371, #12943 ), #67891, .F. ) ;
#16709=CARTESIAN_POINT ( 'NONE',  ( 242.3160000000000025, 65.43750000000000000, -63.94449999999999790 ) ) ;
#16767=CARTESIAN_POINT ( 'NONE',  ( 210.2301280605339855, 25.81350000000000477, -7.937500000000000000 ) ) ;
#16889=EDGE_CURVE ( 'NONE', #46304, #54672, #49770, .T. ) ;
#16909=VECTOR ( 'NONE', #53092, 1000.000000000000000 ) ;
#16914=ADVANCED_FACE ( 'NONE', ( #14283 ), #41957, .T. ) ;
#16922=DIRECTION ( 'NONE',  ( 0.000000000000000000, 0.000000000000000000, 1.000000000000000000 ) ) ;
#17038=CARTESIAN_POINT ( 'NONE',  ( 183.5150000000000148, 52.73749999999999716, -62.78087104677060637 ) ) ;
#17039=DIRECTION ( 'NONE',  ( 0.000000000000000000, 0.000000000000000000, 1.000000000000000000 ) ) ;
#17074=ADVANCED_FACE ( 'NONE', ( #4921 ), #87155, .T. ) ;
#17082=CARTESIAN_POINT ( 'NONE',  ( 210.5660000000000025, 52.73749999999999716, -44.45000000000000284 ) ) ;
#17091=ORIENTED_EDGE ( 'NONE', *, *, #46147, .F. ) ;
#17152=VECTOR ( 'NONE', #15087, 1000.000000000000000 ) ;
#17157=ADVANCED_FACE ( 'NONE', ( #39872 ), #13087, .F. ) ;
#17174=ORIENTED_EDGE ( 'NONE', *, *, #77090, .F. ) ;
#17179=FACE_OUTER_BOUND ( 'NONE', #20857, .T. ) ;
#17246=CARTESIAN_POINT ( 'NONE',  ( 219.9639999999999986, 40.03750000000000142, -58.73749999999999716 ) ) ;
#17281=VECTOR ( 'NONE', #42233, 1000.000000000000000 ) ;
#17285=CIRCLE ( 'NONE', #72400, 8.928099999999993486 ) ;
#17314=CARTESIAN_POINT ( 'NONE',  ( 173.9900000000000091, 5.112500000000000711, -7.937500000000000000 ) ) ;
#17321=DIRECTION ( 'NONE',  ( 1.000000000000000000, 0.000000000000000000, 0.000000000000000000 ) ) ;
#17347=DIRECTION ( 'NONE',  ( 1.000000000000000000, -2.098553464303459752E-16, 0.000000000000000000 ) ) ;
#17373=CARTESIAN_POINT ( 'NONE',  ( 70.98999999999998067, 52.73749999999999716, -44.45000000000002416 ) ) ;
#17425=ORIENTED_EDGE ( 'NONE', *, *, #65942, .F. ) ;
#17482=VECTOR ( 'NONE', #25594, 1000.000000000000000 ) ;
#17519=ORIENTED_EDGE ( 'NONE', *, *, #78101, .F. ) ;
#17558=AXIS2_PLACEMENT_3D ( 'NONE', #46350, #52702, #17778 ) ;
#17568=CARTESIAN_POINT ( 'NONE',  ( 213.4642805167760002, 52.73749999999999716, -54.26046066215670294 ) ) ;
#17664=LINE ( 'NONE', #23166, #59895 ) ;
#17714=DIRECTION ( 'NONE',  ( 0.000000000000000000, 3.785359618865284342E-16, -1.000000000000000000 ) ) ;
#17722=EDGE_LOOP ( 'NONE', ( #29195, #59870, #40794, #35210 ) ) ;
#17755=LINE ( 'NONE', #19535, #16012 ) ;
#17778=DIRECTION ( 'NONE',  ( 0.000000000000000000, 0.000000000000000000, 1.000000000000000000 ) ) ;
#17786=FACE_OUTER_BOUND ( 'NONE', #62534, .T. ) ;
#17799=EDGE_CURVE ( 'NONE', #30283, #18647, #69759, .T. ) ;
#17812=SURFACE_SIDE_STYLE ('',( #87307 ) ) ;
#17830=DIRECTION ( 'NONE',  ( 0.000000000000000000, 0.000000000000000000, -1.000000000000000000 ) ) ;
#17907=CARTESIAN_POINT ( 'NONE',  ( 270.8910000000000196, 65.43750000000000000, -67.11950000000000216 ) ) ;
#17912=LINE ( 'NONE', #16152, #82574 ) ;
#17923=CARTESIAN_POINT ( 'NONE',  ( 245.4909999999999854, 40.03750000000000142, -67.11950000000000216 ) ) ;
#17931=DIRECTION ( 'NONE',  ( -1.000000000000000000, 0.000000000000000000, 0.000000000000000000 ) ) ;
#17961=CARTESIAN_POINT ( 'NONE',  ( 199.3900000000000148, 59.08750000000000568, -38.10000000000000142 ) ) ;
#17992=VERTEX_POINT ( 'NONE', #24 ) ;
#18033=ORIENTED_EDGE ( 'NONE', *, *, #65451, .T. ) ;
#18063=DIRECTION ( 'NONE',  ( 0.000000000000000000, 5.463695987328529395E-16, -1.000000000000000000 ) ) ;
#18133=PLANE ( 'NONE',  #78556 ) ;
#18179=DIRECTION ( 'NONE',  ( 0.000000000000000000, 0.000000000000000000, -1.000000000000000000 ) ) ;
#18182=CIRCLE ( 'NONE', #86352, 10.66799999999999748 ) ;
#18201=EDGE_CURVE ( 'NONE', #69678, #26649, #32630, .T. ) ;
#18218=EDGE_CURVE ( 'NONE', #2953, #22107, #62553, .T. ) ;
#18256=PLANE ( 'NONE',  #55015 ) ;
#18328=CARTESIAN_POINT ( 'NONE',  ( 173.9900000000000091, 36.86249999999999716, -53.61543552338530105 ) ) ;
#18365=PLANE ( 'NONE',  #2427 ) ;
#18375=CIRCLE ( 'NONE', #35750, 4.762500000000001066 ) ;
#18398=CARTESIAN_POINT ( 'NONE',  ( 204.2160000000000082, 52.73749999999999716, -44.45000000000000284 ) ) ;
#18521=DIRECTION ( 'NONE',  ( -1.000000000000000000, 0.000000000000000000, 0.000000000000000000 ) ) ;
#18647=VERTEX_POINT ( 'NONE', #24387 ) ;
#18675=DIRECTION ( 'NONE',  ( 1.000000000000000000, -2.098553464303459752E-16, 0.000000000000000000 ) ) ;
#18678=CIRCLE ( 'NONE', #47647, 9.524999999999998579 ) ;
#18747=DIRECTION ( 'NONE',  ( 1.000000000000000000, 0.000000000000000000, 0.000000000000000000 ) ) ;
#18772=ORIENTED_EDGE ( 'NONE', *, *, #21719, .F. ) ;
#18782=DIRECTION ( 'NONE',  ( 0.000000000000000000, 0.8660254037844387076, -0.4999999999999998890 ) ) ;
#18804=AXIS2_PLACEMENT_3D ( 'NONE', #48352, #89736, #14323 ) ;
#18819=VECTOR ( 'NONE', #15302, 1000.000000000000000 ) ;
#18889=CARTESIAN_POINT ( 'NONE',  ( 173.9900000000000091, 5.112500000000000711, -7.937500000000000000 ) ) ;
#18949=VERTEX_POINT ( 'NONE', #67732 ) ;
#19031=ORIENTED_EDGE ( 'NONE', *, *, #70012, .F. ) ;
#19134=PLANE ( 'NONE',  #41575 ) ;
#19138=DIRECTION ( 'NONE',  ( 1.000000000000000000, 0.000000000000000000, 0.000000000000000000 ) ) ;
#19148=AXIS2_PLACEMENT_3D ( 'NONE', #50988, #58255, #78729 ) ;
#19265=DIRECTION ( 'NONE',  ( 0.000000000000000000, 0.000000000000000000, 1.000000000000000000 ) ) ;
#19301=DIRECTION ( 'NONE',  ( 0.000000000000000000, 0.000000000000000000, -1.000000000000000000 ) ) ;
#19360=ORIENTED_EDGE ( 'NONE', *, *, #41587, .T. ) ;
#19388=FACE_OUTER_BOUND ( 'NONE', #84022, .T. ) ;
#19482=CARTESIAN_POINT ( 'NONE',  ( 70.98999999999998067, 52.73749999999999716, -44.45000000000002416 ) ) ;
#19535=CARTESIAN_POINT ( 'NONE',  ( 226.4410000000000025, 65.43750000000000000, -2.032000000000000028 ) ) ;
#19638=CARTESIAN_POINT ( 'NONE',  ( 177.1649999999999920, 25.81350000000000477, -58.73749999999999716 ) ) ;
#19677=VERTEX_POINT ( 'NONE', #20820 ) ;
#19735=ORIENTED_EDGE ( 'NONE', *, *, #16518, .F. ) ;
#19750=ORIENTED_EDGE ( 'NONE', *, *, #25941, .F. ) ;
#19826=CARTESIAN_POINT ( 'NONE',  ( 226.4410000000000025, 40.03750000000000142, 10.66800000000000104 ) ) ;
#19847=EDGE_CURVE ( 'NONE', #72244, #59868, #85755, .T. ) ;
#19857=EDGE_LOOP ( 'NONE', ( #37642, #36610, #30655, #41023, #19031, #85076 ) ) ;
#19863=DIRECTION ( 'NONE',  ( 1.151873470568221791E-31, -1.000000000000000000, -5.463695987328529395E-16 ) ) ;
#19894=DIRECTION ( 'NONE',  ( 0.000000000000000000, -1.000000000000000000, 0.000000000000000000 ) ) ;
#19900=VERTEX_POINT ( 'NONE', #43478 ) ;
#19983=ORIENTED_EDGE ( 'NONE', *, *, #65709, .T. ) ;
#20056=ORIENTED_EDGE ( 'NONE', *, *, #33572, .F. ) ;
#20059=FACE_OUTER_BOUND ( 'NONE', #20874, .T. ) ;
#20070=FACE_OUTER_BOUND ( 'NONE', #44945, .T. ) ;
#20110=ORIENTED_EDGE ( 'NONE', *, *, #11891, .F. ) ;
#20133=DIRECTION ( 'NONE',  ( 0.7071067811865344721, 0.000000000000000000, -0.7071067811865604513 ) ) ;
#20177=ORIENTED_EDGE ( 'NONE', *, *, #68762, .T. ) ;
#20244=ORIENTED_EDGE ( 'NONE', *, *, #739, .F. ) ;
#20438=EDGE_CURVE ( 'NONE', #28826, #30158, #79806, .T. ) ;
#20528=DIRECTION ( 'NONE',  ( 0.000000000000000000, 0.000000000000000000, -1.000000000000000000 ) ) ;
#20538=DIRECTION ( 'NONE',  ( -1.000000000000000000, 0.000000000000000000, 0.000000000000000000 ) ) ;
#20601=AXIS2_PLACEMENT_3D ( 'NONE', #75808, #47178, #61269 ) ;
#20634=VECTOR ( 'NONE', #86619, 1000.000000000000000 ) ;
#20686=ORIENTED_EDGE ( 'NONE', *, *, #739, .T. ) ;
#20820=CARTESIAN_POINT ( 'NONE',  ( 183.5150000000000148, 14.63749999999999929, -19.05000000000000071 ) ) ;
#20857=EDGE_LOOP ( 'NONE', ( #24503, #41992, #43822, #49207, #19735, #60700 ) ) ;
#20874=EDGE_LOOP ( 'NONE', ( #59520, #45755, #35073, #15191 ) ) ;
#20936=VERTEX_POINT ( 'NONE', #82486 ) ;
#20980=DIRECTION ( 'NONE',  ( 0.000000000000000000, 0.000000000000000000, -1.000000000000000000 ) ) ;
#21006=LINE ( 'NONE', #61874, #47648 ) ;
#21071=DIRECTION ( 'NONE',  ( 0.000000000000000000, -1.000000000000000000, 5.463695987328529395E-16 ) ) ;
#21120=AXIS2_PLACEMENT_3D ( 'NONE', #41284, #28109, #75388 ) ;
#21150=CARTESIAN_POINT ( 'NONE',  ( 204.2160000000000082, 52.73749999999999716, -44.45000000000000284 ) ) ;
#21189=CARTESIAN_POINT ( 'NONE',  ( 208.9149999999999920, 28.98850000000000193, -7.937500000000000000 ) ) ;
#21202=EDGE_CURVE ( 'NONE', #84828, #55699, #66932, .T. ) ;
#21214=CARTESIAN_POINT ( 'NONE',  ( 173.9900000000000091, 5.112500000000000711, -58.73749999999999716 ) ) ;
#21226=LINE ( 'NONE', #70725, #3249 ) ;
#21263=EDGE_CURVE ( 'NONE', #64803, #11195, #52803, .T. ) ;
#21317=CARTESIAN_POINT ( 'NONE',  ( 221.2791280605339921, 36.86249999999999716, -7.937500000000000000 ) ) ;
#21377=CIRCLE ( 'NONE', #40217, 10.26166025953212468 ) ;
#21388=FACE_OUTER_BOUND ( 'NONE', #72096, .T. ) ;
#21394=ADVANCED_FACE ( 'NONE', ( #89174 ), #28733, .T. ) ;
#21495=CARTESIAN_POINT ( 'NONE',  ( 274.0659999999999741, 36.86249999999999716, -58.73749999999999716 ) ) ;
#21518=EDGE_CURVE ( 'NONE', #13566, #64462, #58652, .T. ) ;
#21545=LINE ( 'NONE', #80527, #12402 ) ;
#21646=DIRECTION ( 'NONE',  ( 0.000000000000000000, -1.000000000000000000, 0.000000000000000000 ) ) ;
#21665=ORIENTED_EDGE ( 'NONE', *, *, #84795, .T. ) ;
#21668=VERTEX_POINT ( 'NONE', #11871 ) ;
#21719=EDGE_CURVE ( 'NONE', #44015, #42989, #5049, .T. ) ;
#21835=CARTESIAN_POINT ( 'NONE',  ( 183.5150000000000148, 14.63749999999999929, -19.05000000000000071 ) ) ;
#21859=ORIENTED_EDGE ( 'NONE', *, *, #73569, .F. ) ;
#21866=ORIENTED_EDGE ( 'NONE', *, *, #11891, .T. ) ;
#21897=DIRECTION ( 'NONE',  ( 0.000000000000000000, -1.000000000000000000, 0.000000000000000000 ) ) ;
#22077=EDGE_LOOP ( 'NONE', ( #35166, #53840, #81951, #38348 ) ) ;
#22102=CARTESIAN_POINT ( 'NONE',  ( 199.3900000000000148, 52.73749999999999716, -34.92499999999999716 ) ) ;
#22107=VERTEX_POINT ( 'NONE', #32185 ) ;
#22124=CARTESIAN_POINT ( 'NONE',  ( 226.4410000000000025, 40.03750000000000142, -58.73749999999999716 ) ) ;
#22159=AXIS2_PLACEMENT_3D ( 'NONE', #59380, #25317, #4881 ) ;
#22247=ORIENTED_EDGE ( 'NONE', *, *, #38084, .T. ) ;
#22249=DIRECTION ( 'NONE',  ( 1.000000000000000000, 0.000000000000000000, 3.902639990948949304E-17 ) ) ;
#22330=CARTESIAN_POINT ( 'NONE',  ( 245.4909999999999854, 65.43750000000000000, -67.11950000000000216 ) ) ;
#22734=CONICAL_SURFACE ( 'NONE', #80688, 3.968750000000520473, 0.7853981633974667087 ) ;
#22830=ORIENTED_EDGE ( 'NONE', *, *, #29741, .T. ) ;
#22882=VECTOR ( 'NONE', #18063, 1000.000000000000000 ) ;
#22950=EDGE_LOOP ( 'NONE', ( #2031, #85623, #66938, #80674 ) ) ;
#22994=DIRECTION ( 'NONE',  ( -1.000000000000000000, 0.000000000000000000, -2.108231265501709878E-16 ) ) ;
#23000=EDGE_LOOP ( 'NONE', ( #53611, #75190 ) ) ;
#23004=LINE ( 'NONE', #72910, #80713 ) ;
#23105=EDGE_CURVE ( 'NONE', #18949, #19900, #48169, .T. ) ;
#23166=CARTESIAN_POINT ( 'NONE',  ( 183.5150000000000148, 52.73749999999999716, -26.11912895322935313 ) ) ;
#23173=FACE_OUTER_BOUND ( 'NONE', #43292, .T. ) ;
#23184=CARTESIAN_POINT ( 'NONE',  ( 204.2160000000000082, 52.73749999999999716, -44.45000000000000284 ) ) ;
#23261=DIRECTION ( 'NONE',  ( -0.000000000000000000, 1.000000000000000000, 0.000000000000000000 ) ) ;
#23264=EDGE_CURVE ( 'NONE', #6675, #15555, #57233, .T. ) ;
#23279=EDGE_CURVE ( 'NONE', #10350, #54390, #6480, .T. ) ;
#23344=ORIENTED_EDGE ( 'NONE', *, *, #84795, .F. ) ;
#23516=CARTESIAN_POINT ( 'NONE',  ( 213.1962561210690126, 52.73749999999999716, -41.27499999999999858 ) ) ;
#23574=CARTESIAN_POINT ( 'NONE',  ( 173.9900000000000091, 28.98850000000000193, -58.73749999999999716 ) ) ;
#23601=EDGE_CURVE ( 'NONE', #2953, #28826, #15816, .T. ) ;
#23610=CARTESIAN_POINT ( 'NONE',  ( 199.3900000000000148, 52.73749999999999716, -44.45000000000000284 ) ) ;
#23624=FILL_AREA_STYLE ('',( #36791 ) ) ;
#23673=ADVANCED_FACE ( 'NONE', ( #77146, #29440 ), #832, .T. ) ;
#23726=DIRECTION ( 'NONE',  ( 0.000000000000000000, 0.8660254037844387076, -0.4999999999999998890 ) ) ;
#23756=ADVANCED_FACE ( 'NONE', ( #80723 ), #53415, .T. ) ;
#23849=ORIENTED_EDGE ( 'NONE', *, *, #76693, .T. ) ;
#23865=FACE_OUTER_BOUND ( 'NONE', #46263, .T. ) ;
#23984=CARTESIAN_POINT ( 'NONE',  ( 221.2791280605339921, 36.86249999999999716, -58.73749999999999716 ) ) ;
#24004=ORIENTED_EDGE ( 'NONE', *, *, #18218, .F. ) ;
#24022=ADVANCED_FACE ( 'NONE', ( #61154, #27532 ), #34792, .T. ) ;
#24064=LINE ( 'NONE', #17246, #6839 ) ;
#24078=ORIENTED_EDGE ( 'NONE', *, *, #59651, .F. ) ;
#24080=DIRECTION ( 'NONE',  ( 0.000000000000000000, 0.000000000000000000, -1.000000000000000000 ) ) ;
#24110=AXIS2_PLACEMENT_3D ( 'NONE', #43408, #64327, #42510 ) ;
#24264=AXIS2_PLACEMENT_3D ( 'NONE', #8455, #36153, #63869 ) ;
#24318=FACE_OUTER_BOUND ( 'NONE', #63090, .T. ) ;
#24361=ADVANCED_FACE ( 'NONE', ( #66967 ), #87866, .T. ) ;
#24386=( NAMED_UNIT ( * ) SI_UNIT ( $, .STERADIAN. ) SOLID_ANGLE_UNIT ( ) );
#24387=CARTESIAN_POINT ( 'NONE',  ( 177.1649999999999920, 14.63749999999999929, -19.05000000000000071 ) ) ;
#24503=ORIENTED_EDGE ( 'NONE', *, *, #85741, .F. ) ;
#24584=DIRECTION ( 'NONE',  ( 5.463695987328529395E-16, 0.000000000000000000, 1.000000000000000000 ) ) ;
#24590=EDGE_LOOP ( 'NONE', ( #37389, #8938, #34486, #81597 ) ) ;
#24639=DIRECTION ( 'NONE',  ( -0.5000000000000003331, 0.8660254037844383745, 0.000000000000000000 ) ) ;
#24807=DIRECTION ( 'NONE',  ( 3.902639990948949304E-17, 0.000000000000000000, -1.000000000000000000 ) ) ;
#24899=VERTEX_POINT ( 'NONE', #63133 ) ;
#24925=EDGE_LOOP ( 'NONE', ( #51818, #76708, #50378, #4819 ) ) ;
#25005=VERTEX_POINT ( 'NONE', #18889 ) ;
#25083=DIRECTION ( 'NONE',  ( 1.000000000000000000, 0.000000000000000000, 0.000000000000000000 ) ) ;
#25134=VERTEX_POINT ( 'NONE', #52478 ) ;
#25214=EDGE_LOOP ( 'NONE', ( #52105, #27194 ) ) ;
#25276=DIRECTION ( 'NONE',  ( 0.000000000000000000, 0.000000000000000000, 1.000000000000000000 ) ) ;
#25308=ORIENTED_EDGE ( 'NONE', *, *, #23105, .F. ) ;
#25317=DIRECTION ( 'NONE',  ( 1.000000000000000000, 0.000000000000000000, 0.000000000000000000 ) ) ;
#25383=DIRECTION ( 'NONE',  ( -1.000000000000000000, 0.000000000000000000, 0.000000000000000000 ) ) ;
#25414=SHAPE_DEFINITION_REPRESENTATION ( #88094, #47290 ) ;
#25420=CARTESIAN_POINT ( 'NONE',  ( 274.0659999999999741, 36.86249999999999716, -7.937500000000000000 ) ) ;
#25495=ORIENTED_EDGE ( 'NONE', *, *, #65670, .F. ) ;
#25587=EDGE_CURVE ( 'NONE', #42451, #31104, #56426, .T. ) ;
#25594=DIRECTION ( 'NONE',  ( 1.000000000000000000, 0.000000000000000000, 2.108231265501709878E-16 ) ) ;
#25602=ADVANCED_FACE ( 'NONE', ( #77338, #8302 ), #8761, .T. ) ;
#25609=LINE ( 'NONE', #75105, #3078 ) ;
#25610=CARTESIAN_POINT ( 'NONE',  ( 223.2659999999999911, 52.73749999999999716, -33.78199999999999648 ) ) ;
#25622=TOROIDAL_SURFACE ( 'NONE', #25686, 6.647542495715439870, 3.174999999999999822 ) ;
#25630=CARTESIAN_POINT ( 'NONE',  ( 199.3900000000000148, 52.73749999999999716, -44.45000000000000284 ) ) ;
#25678=CARTESIAN_POINT ( 'NONE',  ( 270.8910000000000196, 65.43750000000000000, -67.11950000000000216 ) ) ;
#25686=AXIS2_PLACEMENT_3D ( 'NONE', #31157, #84374, #43892 ) ;
#25767=VECTOR ( 'NONE', #87072, 1000.000000000000000 ) ;
#25770=EDGE_LOOP ( 'NONE', ( #11404, #48331 ) ) ;
#25876=LINE ( 'NONE', #3643, #16909 ) ;
#25941=EDGE_CURVE ( 'NONE', #14995, #30543, #15472, .T. ) ;
#26092=ORIENTED_EDGE ( 'NONE', *, *, #53450, .T. ) ;
#26117=LINE ( 'NONE', #74269, #14268 ) ;
#26176=LINE ( 'NONE', #13006, #54664 ) ;
#26294=ORIENTED_EDGE ( 'NONE', *, *, #89339, .T. ) ;
#26306=DIRECTION ( 'NONE',  ( 0.000000000000000000, 0.000000000000000000, -1.000000000000000000 ) ) ;
#26309=DIRECTION ( 'NONE',  ( -7.136255983449500255E-16, 0.000000000000000000, -1.000000000000000000 ) ) ;
#26344=FACE_OUTER_BOUND ( 'NONE', #29105, .T. ) ;
#26459=DIRECTION ( 'NONE',  ( 0.000000000000000000, 3.785359618865284342E-16, -1.000000000000000000 ) ) ;
#26604=AXIS2_PLACEMENT_3D ( 'NONE', #45963, #60497, #66877 ) ;
#26630=CARTESIAN_POINT ( 'NONE',  ( 239.7378999999999962, 52.73749999999999716, 10.66800000000000104 ) ) ;
#26632=ADVANCED_FACE ( 'NONE', ( #65284 ), #51633, .T. ) ;
#26634=DIRECTION ( 'NONE',  ( 0.000000000000000000, 0.000000000000000000, 1.000000000000000000 ) ) ;
#26649=VERTEX_POINT ( 'NONE', #44824 ) ;
#26794=VECTOR ( 'NONE', #83662, 1000.000000000000000 ) ;
#26821=ADVANCED_FACE ( 'NONE', ( #44147 ), #84183, .F. ) ;
#26920=ADVANCED_FACE ( 'NONE', ( #78268 ), #37809, .T. ) ;
#26934=ADVANCED_FACE ( 'NONE', ( #11894 ), #46826, .F. ) ;
#27057=VECTOR ( 'NONE', #16922, 1000.000000000000000 ) ;
#27100=FACE_OUTER_BOUND ( 'NONE', #37064, .T. ) ;
#27101=LINE ( 'NONE', #81640, #89547 ) ;
#27120=ORIENTED_EDGE ( 'NONE', *, *, #85298, .F. ) ;
#27194=ORIENTED_EDGE ( 'NONE', *, *, #55904, .F. ) ;
#27230=DIRECTION ( 'NONE',  ( 0.000000000000000000, -1.000000000000000000, 0.000000000000000000 ) ) ;
#27240=DIRECTION ( 'NONE',  ( -1.000000000000000000, 0.000000000000000000, -2.108231265501709878E-16 ) ) ;
#27257=TOROIDAL_SURFACE ( 'NONE', #63575, 6.647542495715439870, 3.174999999999999822 ) ;
#27329=ORIENTED_EDGE ( 'NONE', *, *, #5664, .T. ) ;
#27335=CARTESIAN_POINT ( 'NONE',  ( 223.2659999999999911, 52.73749999999999716, -44.45000000000000284 ) ) ;
#27368=LINE ( 'NONE', #81468, #78954 ) ;
#27434=AXIS2_PLACEMENT_3D ( 'NONE', #29474, #35372, #63084 ) ;
#27532=FACE_BOUND ( 'NONE', #17722, .T. ) ;
#27607=VECTOR ( 'NONE', #27240, 1000.000000000000000 ) ;
#27618=CIRCLE ( 'NONE', #82762, 4.762500000000002842 ) ;
#27620=EDGE_CURVE ( 'NONE', #25005, #40315, #81300, .T. ) ;
#27749=CARTESIAN_POINT ( 'NONE',  ( 219.9639999999999986, 40.03750000000000142, -7.937500000000000000 ) ) ;
#27967=DIRECTION ( 'NONE',  ( -1.000000000000000000, 0.000000000000000000, 0.000000000000000000 ) ) ;
#27998=ORIENTED_EDGE ( 'NONE', *, *, #64168, .T. ) ;
#28009=LINE ( 'NONE', #62979, #18819 ) ;
#28012=DIRECTION ( 'NONE',  ( 0.000000000000000000, -1.000000000000000000, 0.000000000000000000 ) ) ;
#28074=DIRECTION ( 'NONE',  ( 0.000000000000000000, 1.000000000000000000, 0.000000000000000000 ) ) ;
#28109=DIRECTION ( 'NONE',  ( 1.000000000000000000, 0.000000000000000000, 0.000000000000000000 ) ) ;
#28122=VECTOR ( 'NONE', #33668, 1000.000000000000000 ) ;
#28172=DIRECTION ( 'NONE',  ( 0.000000000000000000, 0.8660254037844387076, 0.4999999999999998890 ) ) ;
#28210=ADVANCED_FACE ( 'NONE', ( #29345 ), #1645, .F. ) ;
#28220=VECTOR ( 'NONE', #29581, 1000.000000000000000 ) ;
#28239=PLANE ( 'NONE',  #32819 ) ;
#28257=ORIENTED_EDGE ( 'NONE', *, *, #73569, .T. ) ;
#28267=ORIENTED_EDGE ( 'NONE', *, *, #33572, .T. ) ;
#28353=ADVANCED_FACE ( 'NONE', ( #57480 ), #7994, .F. ) ;
#28430=DIRECTION ( 'NONE',  ( 0.000000000000000000, -1.000000000000000000, 0.000000000000000000 ) ) ;
#28475=AXIS2_PLACEMENT_3D ( 'NONE', #45481, #52729, #50977 ) ;
#28479=ORIENTED_EDGE ( 'NONE', *, *, #35304, .T. ) ;
#28522=CARTESIAN_POINT ( 'NONE',  ( 199.3900000000000148, 52.73749999999999716, -44.45000000000000284 ) ) ;
#28543=EDGE_CURVE ( 'NONE', #82635, #37523, #74683, .T. ) ;
#28585=CARTESIAN_POINT ( 'NONE',  ( 186.6899999999999977, 52.73749999999999716, -34.92499999999999716 ) ) ;
#28622=VERTEX_POINT ( 'NONE', #56918 ) ;
#28632=DIRECTION ( 'NONE',  ( 0.000000000000000000, 1.000000000000000000, 0.000000000000000000 ) ) ;
#28733=PLANE ( 'NONE',  #87185 ) ;
#28762=UNCERTAINTY_MEASURE_WITH_UNIT (LENGTH_MEASURE( 1.000000000000000082E-05 ), #3736, 'distance_accuracy_value', 'NONE');
#28792=EDGE_CURVE ( 'NONE', #10845, #25134, #36931, .T. ) ;
#28798=CARTESIAN_POINT ( 'NONE',  ( 70.98999999999998067, 52.73749999999999716, -36.61250000000002558 ) ) ;
#28807=CARTESIAN_POINT ( 'NONE',  ( 223.2659999999999911, 52.73749999999999716, -44.45000000000000284 ) ) ;
#28826=VERTEX_POINT ( 'NONE', #74474 ) ;
#28832=FACE_OUTER_BOUND ( 'NONE', #87241, .T. ) ;
#28851=EDGE_LOOP ( 'NONE', ( #74316, #48845 ) ) ;
#28853=ADVANCED_FACE ( 'NONE', ( #16493 ), #80857, .F. ) ;
#28876=FACE_OUTER_BOUND ( 'NONE', #59902, .T. ) ;
#28904=CARTESIAN_POINT ( 'NONE',  ( 242.3160000000000025, 65.43750000000000000, -63.94449999999999790 ) ) ;
#28996=ORIENTED_EDGE ( 'NONE', *, *, #50798, .F. ) ;
#29072=ORIENTED_EDGE ( 'NONE', *, *, #23601, .T. ) ;
#29105=EDGE_LOOP ( 'NONE', ( #81992, #84810, #66999, #65600, #7063, #55947, #8461, #80638, #46218, #76295 ) ) ;
#29195=ORIENTED_EDGE ( 'NONE', *, *, #41285, .F. ) ;
#29197=DIRECTION ( 'NONE',  ( -1.000000000000000000, 0.000000000000000000, 0.000000000000000000 ) ) ;
#29220=CARTESIAN_POINT ( 'NONE',  ( 183.5150000000000148, 52.73749999999999716, -26.11912895322935313 ) ) ;
#29242=ORIENTED_EDGE ( 'NONE', *, *, #76047, .F. ) ;
#29265=CARTESIAN_POINT ( 'NONE',  ( 177.1649999999999920, 14.63749999999999929, -9.525000000000000355 ) ) ;
#29296=CARTESIAN_POINT ( 'NONE',  ( 219.9639999999999986, 40.03750000000000142, -7.937500000000000000 ) ) ;
#29336=CARTESIAN_POINT ( 'NONE',  ( 219.9639999999999986, 40.03750000000000142, -7.937500000000000000 ) ) ;
#29345=FACE_OUTER_BOUND ( 'NONE', #24925, .T. ) ;
#29349=CARTESIAN_POINT ( 'NONE',  ( 223.2659999999999911, 52.73749999999999716, -56.89600000000000080 ) ) ;
#29440=FACE_BOUND ( 'NONE', #43952, .T. ) ;
#29474=CARTESIAN_POINT ( 'NONE',  ( 226.4410000000000025, 65.43750000000000000, 10.66800000000000104 ) ) ;
#29517=ORIENTED_EDGE ( 'NONE', *, *, #62372, .F. ) ;
#29579=CARTESIAN_POINT ( 'NONE',  ( 241.3336515812914911, 40.03750000000000142, -2.032000000000000028 ) ) ;
#29581=DIRECTION ( 'NONE',  ( 0.000000000000000000, 0.000000000000000000, 1.000000000000000000 ) ) ;
#29660=CARTESIAN_POINT ( 'NONE',  ( 255.9983484187079910, 40.03750000000000142, 10.66800000000000104 ) ) ;
#29741=EDGE_CURVE ( 'NONE', #73485, #84299, #58841, .T. ) ;
#29821=DIRECTION ( 'NONE',  ( 0.000000000000000000, 0.000000000000000000, 1.000000000000000000 ) ) ;
#29844=CARTESIAN_POINT ( 'NONE',  ( 226.4410000000000025, 40.03750000000000142, -2.032000000000000028 ) ) ;
#29964=DIRECTION ( 'NONE',  ( 0.000000000000000000, -0.8660254037844387076, 0.4999999999999998890 ) ) ;
#30001=CARTESIAN_POINT ( 'NONE',  ( 177.1649999999999920, 14.63749999999999929, -47.62500000000000000 ) ) ;
#30017=ADVANCED_FACE ( 'NONE', ( #69253 ), #68806, .T. ) ;
#30074=DIRECTION ( 'NONE',  ( -1.000000000000000000, 0.000000000000000000, 0.000000000000000000 ) ) ;
#30085=LINE ( 'NONE', #4160, #89458 ) ;
#30094=EDGE_CURVE ( 'NONE', #30425, #46304, #82454, .T. ) ;
#30158=VERTEX_POINT ( 'NONE', #42864 ) ;
#30180=PLANE ( 'NONE',  #88466 ) ;
#30283=VERTEX_POINT ( 'NONE', #29265 ) ;
#30418=DIRECTION ( 'NONE',  ( 0.000000000000000000, -1.000000000000000000, 0.000000000000000000 ) ) ;
#30420=DIRECTION ( 'NONE',  ( 1.000000000000000000, 0.000000000000000000, 0.000000000000000000 ) ) ;
#30425=VERTEX_POINT ( 'NONE', #87794 ) ;
#30447=VERTEX_POINT ( 'NONE', #49905 ) ;
#30527=EDGE_LOOP ( 'NONE', ( #44788, #6841, #35268, #35772, #47034, #8429, #89484, #15633, #82719, #23344, #13321, #19750 ) ) ;
#30543=VERTEX_POINT ( 'NONE', #16308 ) ;
#30544=CARTESIAN_POINT ( 'NONE',  ( 173.9900000000000091, 14.32000000000000028, -71.37400000000000944 ) ) ;
#30550=UNCERTAINTY_MEASURE_WITH_UNIT (LENGTH_MEASURE( 1.000000000000000082E-05 ), #31626, 'distance_accuracy_value', 'NONE');
#30553=SHAPE_REPRESENTATION_RELATIONSHIP ( 'NONE' , 'NONE' ,  #47290, #60825 ) ;
#30655=ORIENTED_EDGE ( 'NONE', *, *, #71368, .T. ) ;
#30720=EDGE_CURVE ( 'NONE', #3831, #31184, #48085, .T. ) ;
#30774=DIRECTION ( 'NONE',  ( 1.000000000000000000, 0.000000000000000000, -0.000000000000000000 ) ) ;
#30861=AXIS2_PLACEMENT_3D ( 'NONE', #76524, #83800, #83347 ) ;
#30920=EDGE_CURVE ( 'NONE', #71852, #8565, #21226, .T. ) ;
#30924=ORIENTED_EDGE ( 'NONE', *, *, #41066, .T. ) ;
#30956=VECTOR ( 'NONE', #14163, 1000.000000000000000 ) ;
#30973=CYLINDRICAL_SURFACE ( 'NONE', #32670, 4.762500000000002842 ) ;
#30982=DIRECTION ( 'NONE',  ( 2.108231265501709878E-16, 0.000000000000000000, -1.000000000000000000 ) ) ;
#30986=EDGE_CURVE ( 'NONE', #13566, #64803, #87031, .T. ) ;
#31104=VERTEX_POINT ( 'NONE', #44328 ) ;
#31129=CARTESIAN_POINT ( 'NONE',  ( 248.6659999999999968, 52.73749999999999716, -2.903194600000015502 ) ) ;
#31157=CARTESIAN_POINT ( 'NONE',  ( 213.7409999999999854, 52.73749999999999716, -44.45000000000000284 ) ) ;
#31184=VERTEX_POINT ( 'NONE', #74735 ) ;
#31249=ORIENTED_EDGE ( 'NONE', *, *, #20438, .F. ) ;
#31261=AXIS2_PLACEMENT_3D ( 'NONE', #44288, #37499, #86104 ) ;
#31288=DIRECTION ( 'NONE',  ( 1.000000000000000000, 0.000000000000000000, 0.000000000000000000 ) ) ;
#31313=EDGE_CURVE ( 'NONE', #74351, #54782, #73384, .T. ) ;
#31319=ADVANCED_FACE ( 'NONE', ( #28832 ), #63344, .F. ) ;
#31531=EDGE_CURVE ( 'NONE', #55564, #65795, #16539, .T. ) ;
#31565=ORIENTED_EDGE ( 'NONE', *, *, #74108, .T. ) ;
#31620=ORIENTED_EDGE ( 'NONE', *, *, #4489, .T. ) ;
#31626=( LENGTH_UNIT ( ) NAMED_UNIT ( * ) SI_UNIT ( .MILLI., .METRE. ) );
#31636=ORIENTED_EDGE ( 'NONE', *, *, #50908, .F. ) ;
#31710=DIRECTION ( 'NONE',  ( -0.4999999999999998890, -0.8660254037844387076, 0.000000000000000000 ) ) ;
#31718=EDGE_LOOP ( 'NONE', ( #50907, #74424, #75937, #19983 ) ) ;
#31726=DIRECTION ( 'NONE',  ( 1.000000000000000000, 0.000000000000000000, 0.000000000000000000 ) ) ;
#31789=STYLED_ITEM ( 'NONE', ( #16040 ), #60825 ) ;
#31794=FACE_BOUND ( 'NONE', #25214, .T. ) ;
#31867=EDGE_CURVE ( 'NONE', #87914, #42451, #21006, .T. ) ;
#31914=ORIENTED_EDGE ( 'NONE', *, *, #33050, .T. ) ;
#31934=ADVANCED_FACE ( 'NONE', ( #82356 ), #79588, .F. ) ;
#31948=ORIENTED_EDGE ( 'NONE', *, *, #54791, .T. ) ;
#31972=DIRECTION ( 'NONE',  ( 0.000000000000000000, 0.000000000000000000, -1.000000000000000000 ) ) ;
#32075=DIRECTION ( 'NONE',  ( 0.000000000000000000, 0.000000000000000000, 1.000000000000000000 ) ) ;
#32098=ORIENTED_EDGE ( 'NONE', *, *, #10919, .T. ) ;
#32119=CIRCLE ( 'NONE', #61173, 7.837499999999996803 ) ;
#32139=CARTESIAN_POINT ( 'NONE',  ( 183.5150000000000148, 36.86249999999999716, -35.28456447661465489 ) ) ;
#32185=CARTESIAN_POINT ( 'NONE',  ( 239.7378999999999962, 52.73749999999999716, -10.97647784993501396 ) ) ;
#32186=VECTOR ( 'NONE', #17714, 1000.000000000000000 ) ;
#32204=DIRECTION ( 'NONE',  ( -0.4999999999999998890, 0.8660254037844387076, 0.000000000000000000 ) ) ;
#32320=DIRECTION ( 'NONE',  ( 1.000000000000000000, 3.651563665954199690E-16, 0.000000000000000000 ) ) ;
#32417=DIRECTION ( 'NONE',  ( 0.000000000000000000, 0.000000000000000000, 1.000000000000000000 ) ) ;
#32452=ORIENTED_EDGE ( 'NONE', *, *, #66428, .F. ) ;
#32482=ADVANCED_FACE ( 'NONE', ( #45662, #1356 ), #56748, .F. ) ;
#32521=DIRECTION ( 'NONE',  ( -0.7071067811865470176, -0.7071067811865480168, 0.000000000000000000 ) ) ;
#32537=DIRECTION ( 'NONE',  ( 0.000000000000000000, 0.000000000000000000, 1.000000000000000000 ) ) ;
#32559=AXIS2_PLACEMENT_3D ( 'NONE', #11465, #89116, #20528 ) ;
#32567=ORIENTED_EDGE ( 'NONE', *, *, #6491, .T. ) ;
#32585=DIRECTION ( 'NONE',  ( 0.000000000000000000, 3.785359618865284342E-16, -1.000000000000000000 ) ) ;
#32630=LINE ( 'NONE', #45795, #46576 ) ;
#32670=AXIS2_PLACEMENT_3D ( 'NONE', #21150, #48822, #77012 ) ;
#32681=ORIENTED_EDGE ( 'NONE', *, *, #66602, .F. ) ;
#32738=ORIENTED_EDGE ( 'NONE', *, *, #29741, .F. ) ;
#32744=PRODUCT_DEFINITION ( 'UNKNOWN', '', #78373, #85085 ) ;
#32802=CARTESIAN_POINT ( 'NONE',  ( 186.6899999999999977, 46.38749999999999574, -50.79999999999999716 ) ) ;
#32816=AXIS2_PLACEMENT_3D ( 'NONE', #25678, #44326, #51585 ) ;
#32819=AXIS2_PLACEMENT_3D ( 'NONE', #49119, #540, #55933 ) ;
#32835=VECTOR ( 'NONE', #61900, 1000.000000000000114 ) ;
#32843=EDGE_LOOP ( 'NONE', ( #86767, #45171 ) ) ;
#32855=VERTEX_POINT ( 'NONE', #41544 ) ;
#32865=CARTESIAN_POINT ( 'NONE',  ( 183.5150000000000148, 14.63749999999999929, -52.38749999999999574 ) ) ;
#32871=LINE ( 'NONE', #4288, #2380 ) ;
#32874=ORIENTED_EDGE ( 'NONE', *, *, #86587, .F. ) ;
#32887=EDGE_CURVE ( 'NONE', #64424, #66028, #46339, .T. ) ;
#32934=DIRECTION ( 'NONE',  ( 0.000000000000000000, 0.000000000000000000, -1.000000000000000000 ) ) ;
#33007=ADVANCED_FACE ( 'NONE', ( #11060 ), #30180, .T. ) ;
#33041=DIRECTION ( 'NONE',  ( 1.000000000000000000, 0.000000000000000000, 0.000000000000000000 ) ) ;
#33047=CARTESIAN_POINT ( 'NONE',  ( 204.2160000000000082, 52.73749999999999716, -44.45000000000000284 ) ) ;
#33050=EDGE_CURVE ( 'NONE', #48266, #82635, #44682, .T. ) ;
#33133=DIRECTION ( 'NONE',  ( 1.000000000000000000, 0.000000000000000000, 0.000000000000000000 ) ) ;
#33205=ORIENTED_EDGE ( 'NONE', *, *, #58850, .T. ) ;
#33206=ORIENTED_EDGE ( 'NONE', *, *, #21518, .T. ) ;
#33313=EDGE_LOOP ( 'NONE', ( #20686, #9061 ) ) ;
#33371=FACE_OUTER_BOUND ( 'NONE', #33313, .T. ) ;
#33443=DIRECTION ( 'NONE',  ( 0.000000000000000000, 0.000000000000000000, 1.000000000000000000 ) ) ;
#33462=DIRECTION ( 'NONE',  ( -1.000000000000000000, 0.000000000000000000, 0.000000000000000000 ) ) ;
#33499=DIRECTION ( 'NONE',  ( 0.000000000000000000, 0.000000000000000000, 1.000000000000000000 ) ) ;
#33520=VECTOR ( 'NONE', #26306, 1000.000000000000000 ) ;
#33553=DIRECTION ( 'NONE',  ( 0.000000000000000000, -0.8660254037844387076, 0.4999999999999998890 ) ) ;
#33554=ORIENTED_EDGE ( 'NONE', *, *, #50908, .T. ) ;
#33572=EDGE_CURVE ( 'NONE', #37178, #30283, #85056, .T. ) ;
#33576=ORIENTED_EDGE ( 'NONE', *, *, #54791, .F. ) ;
#33585=DIRECTION ( 'NONE',  ( 0.000000000000000000, 1.000000000000000000, 0.000000000000000000 ) ) ;
#33594=AXIS2_PLACEMENT_3D ( 'NONE', #88646, #54077, #40022 ) ;
#33605=CARTESIAN_POINT ( 'NONE',  ( 226.4410000000000025, 65.43750000000000000, 10.66800000000000104 ) ) ;
#33614=EDGE_LOOP ( 'NONE', ( #61170, #70355, #6116, #56579, #51631 ) ) ;
#33668=DIRECTION ( 'NONE',  ( 0.000000000000000000, 0.000000000000000000, 1.000000000000000000 ) ) ;
#33684=CARTESIAN_POINT ( 'NONE',  ( 177.1649999999999920, 5.112500000000000711, -7.937500000000000000 ) ) ;
#33795=ADVANCED_FACE ( 'NONE', ( #7290 ), #77228, .F. ) ;
#33801=CARTESIAN_POINT ( 'NONE',  ( 186.6899999999999977, 59.08750000000000568, -38.10000000000000142 ) ) ;
#33911=ORIENTED_EDGE ( 'NONE', *, *, #21719, .T. ) ;
#34049=ORIENTED_EDGE ( 'NONE', *, *, #303, .F. ) ;
#34103=LINE ( 'NONE', #27749, #85332 ) ;
#34110=ORIENTED_EDGE ( 'NONE', *, *, #20438, .T. ) ;
#34113=CIRCLE ( 'NONE', #8009, 7.837499999999996803 ) ;
#34152=CARTESIAN_POINT ( 'NONE',  ( 173.9900000000000091, 36.86249999999999716, -35.28456447661465489 ) ) ;
#34448=ORIENTED_EDGE ( 'NONE', *, *, #6410, .F. ) ;
#34486=ORIENTED_EDGE ( 'NONE', *, *, #28792, .F. ) ;
#34583=DIRECTION ( 'NONE',  ( -1.000000000000000000, 0.000000000000000000, 0.000000000000000000 ) ) ;
#34634=ADVANCED_FACE ( 'NONE', ( #53236 ), #75063, .F. ) ;
#34662=AXIS2_PLACEMENT_3D ( 'NONE', #85590, #44206, #2007 ) ;
#34747=ORIENTED_EDGE ( 'NONE', *, *, #31531, .T. ) ;
#34792=PLANE ( 'NONE',  #83392 ) ;
#34818=VECTOR ( 'NONE', #42499, 1000.000000000000000 ) ;
#34859=ADVANCED_FACE ( 'NONE', ( #50020, #77756 ), #28239, .T. ) ;
#34880=ADVANCED_FACE ( 'NONE', ( #7809 ), #63221, .F. ) ;
#34912=EDGE_LOOP ( 'NONE', ( #67647, #27998 ) ) ;
#34945=DIRECTION ( 'NONE',  ( 0.4999999999999998890, 0.8660254037844387076, 0.000000000000000000 ) ) ;
#34976=DIRECTION ( 'NONE',  ( -1.825781832977093682E-16, -0.5000000000000003331, 0.8660254037844384856 ) ) ;
#35001=ORIENTED_EDGE ( 'NONE', *, *, #18218, .T. ) ;
#35008=VECTOR ( 'NONE', #88778, 1000.000000000000000 ) ;
#35052=DIRECTION ( 'NONE',  ( 0.000000000000000000, 0.000000000000000000, -1.000000000000000000 ) ) ;
#35073=ORIENTED_EDGE ( 'NONE', *, *, #21518, .F. ) ;
#35100=ORIENTED_EDGE ( 'NONE', *, *, #84936, .F. ) ;
#35146=ADVANCED_FACE ( 'NONE', ( #88149 ), #22734, .T. ) ;
#35166=ORIENTED_EDGE ( 'NONE', *, *, #49052, .T. ) ;
#35178=CARTESIAN_POINT ( 'NONE',  ( 183.5150000000000148, 68.61249999999999716, -53.61543552338530105 ) ) ;
#35183=ORIENTED_EDGE ( 'NONE', *, *, #72238, .F. ) ;
#35210=ORIENTED_EDGE ( 'NONE', *, *, #1029, .F. ) ;
#35232=CARTESIAN_POINT ( 'NONE',  ( 242.3160000000000025, 40.03750000000000142, -63.94449999999999790 ) ) ;
#35255=FACE_OUTER_BOUND ( 'NONE', #60492, .T. ) ;
#35265=ORIENTED_EDGE ( 'NONE', *, *, #46147, .T. ) ;
#35268=ORIENTED_EDGE ( 'NONE', *, *, #7485, .F. ) ;
#35275=AXIS2_PLACEMENT_3D ( 'NONE', #56068, #60770, #74864 ) ;
#35304=EDGE_CURVE ( 'NONE', #59900, #84828, #79444, .T. ) ;
#35355=ORIENTED_EDGE ( 'NONE', *, *, #16889, .T. ) ;
#35372=DIRECTION ( 'NONE',  ( 1.000000000000000000, 0.000000000000000000, 0.000000000000000000 ) ) ;
#35497=CARTESIAN_POINT ( 'NONE',  ( 226.4410000000000025, 40.03750000000000142, 10.66800000000000104 ) ) ;
#35513=LINE ( 'NONE', #63689, #60035 ) ;
#35520=ORIENTED_EDGE ( 'NONE', *, *, #52777, .T. ) ;
#35681=DIRECTION ( 'NONE',  ( 0.000000000000000000, 0.000000000000000000, 1.000000000000000000 ) ) ;
#35750=AXIS2_PLACEMENT_3D ( 'NONE', #51390, #16015, #7840 ) ;
#35772=ORIENTED_EDGE ( 'NONE', *, *, #254, .F. ) ;
#35788=DIRECTION ( 'NONE',  ( -2.108231265501709878E-16, 0.000000000000000000, 1.000000000000000000 ) ) ;
#35826=ADVANCED_FACE ( 'NONE', ( #71625 ), #25622, .T. ) ;
#35975=VECTOR ( 'NONE', #21071, 1000.000000000000000 ) ;
#35999=VERTEX_POINT ( 'NONE', #58855 ) ;
#36019=ORIENTED_EDGE ( 'NONE', *, *, #75379, .T. ) ;
#36082=ORIENTED_EDGE ( 'NONE', *, *, #66602, .T. ) ;
#36104=EDGE_CURVE ( 'NONE', #86177, #47225, #7493, .T. ) ;
#36124=ORIENTED_EDGE ( 'NONE', *, *, #65670, .T. ) ;
#36148=ORIENTED_EDGE ( 'NONE', *, *, #48222, .F. ) ;
#36153=DIRECTION ( 'NONE',  ( 0.000000000000000000, 0.000000000000000000, 1.000000000000000000 ) ) ;
#36156=LINE ( 'NONE', #77492, #34818 ) ;
#36166=DIRECTION ( 'NONE',  ( -1.000000000000000000, 0.000000000000000000, 0.000000000000000000 ) ) ;
#36215=ORIENTED_EDGE ( 'NONE', *, *, #62372, .T. ) ;
#36270=ORIENTED_EDGE ( 'NONE', *, *, #36381, .T. ) ;
#36329=DIRECTION ( 'NONE',  ( -1.000000000000000000, 0.000000000000000000, 0.000000000000000000 ) ) ;
#36344=MECHANICAL_DESIGN_GEOMETRIC_PRESENTATION_REPRESENTATION('',(#31789),#78247);
#36347=ORIENTED_EDGE ( 'NONE', *, *, #41285, .T. ) ;
#36367=ORIENTED_EDGE ( 'NONE', *, *, #66428, .T. ) ;
#36381=EDGE_CURVE ( 'NONE', #86672, #64424, #11513, .T. ) ;
#36389=AXIS2_PLACEMENT_3D ( 'NONE', #17082, #44770, #72496 ) ;
#36395=LINE ( 'NONE', #83203, #78424 ) ;
#36610=ORIENTED_EDGE ( 'NONE', *, *, #50798, .T. ) ;
#36611=DIRECTION ( 'NONE',  ( 0.000000000000000000, 0.000000000000000000, -1.000000000000000000 ) ) ;
#36653=AXIS2_PLACEMENT_3D ( 'NONE', #83718, #48715, #6512 ) ;
#36680=CARTESIAN_POINT ( 'NONE',  ( 270.8910000000000196, 40.03750000000000142, -67.11950000000000216 ) ) ;
#36791=FILL_AREA_STYLE_COLOUR ( '', #41278 ) ;
#36807=LINE ( 'NONE', #77699, #81474 ) ;
#36840=CARTESIAN_POINT ( 'NONE',  ( 270.8910000000000196, 65.43750000000000000, -67.11950000000000216 ) ) ;
#36857=LINE ( 'NONE', #50473, #76543 ) ;
#36897=CARTESIAN_POINT ( 'NONE',  ( 204.2160000000000082, 52.73749999999999716, -44.45000000000000284 ) ) ;
#36914=UNCERTAINTY_MEASURE_WITH_UNIT (LENGTH_MEASURE( 1.000000000000000082E-05 ), #36918, 'distance_accuracy_value', 'NONE');
#36918=( LENGTH_UNIT ( ) NAMED_UNIT ( * ) SI_UNIT ( .MILLI., .METRE. ) );
#36931=LINE ( 'NONE', #25420, #42322 ) ;
#37000=ORIENTED_EDGE ( 'NONE', *, *, #54805, .F. ) ;
#37064=EDGE_LOOP ( 'NONE', ( #88055, #9866, #68386, #10290 ) ) ;
#37077=DIRECTION ( 'NONE',  ( 0.000000000000000000, 0.000000000000000000, -1.000000000000000000 ) ) ;
#37178=VERTEX_POINT ( 'NONE', #73400 ) ;
#37190=ORIENTED_EDGE ( 'NONE', *, *, #11535, .T. ) ;
#37261=ORIENTED_EDGE ( 'NONE', *, *, #13599, .T. ) ;
#37365=( NAMED_UNIT ( * ) SI_UNIT ( $, .STERADIAN. ) SOLID_ANGLE_UNIT ( ) );
#37370=FACE_OUTER_BOUND ( 'NONE', #48137, .T. ) ;
#37382=AXIS2_PLACEMENT_3D ( 'NONE', #75062, #68697, #89596 ) ;
#37389=ORIENTED_EDGE ( 'NONE', *, *, #77289, .T. ) ;
#37499=DIRECTION ( 'NONE',  ( -1.000000000000000000, 0.000000000000000000, 0.000000000000000000 ) ) ;
#37523=VERTEX_POINT ( 'NONE', #54011 ) ;
#37529=DIRECTION ( 'NONE',  ( 1.000000000000000000, 0.000000000000000000, 0.000000000000000000 ) ) ;
#37531=DIRECTION ( 'NONE',  ( 0.9961946980917455452, -1.067350013832299363E-17, -0.08715574274765836016 ) ) ;
#37574=AXIS2_PLACEMENT_3D ( 'NONE', #9264, #9707, #38292 ) ;
#37603=ORIENTED_EDGE ( 'NONE', *, *, #1386, .F. ) ;
#37642=ORIENTED_EDGE ( 'NONE', *, *, #19847, .T. ) ;
#37730=CARTESIAN_POINT ( 'NONE',  ( 173.9899999999999807, 52.73749999999999716, -36.61250000000000426 ) ) ;
#37809=CYLINDRICAL_SURFACE ( 'NONE', #68227, 4.762500000000002842 ) ;
#37983=EDGE_CURVE ( 'NONE', #56634, #9037, #64382, .T. ) ;
#38061=VECTOR ( 'NONE', #85266, 1000.000000000000000 ) ;
#38071=CARTESIAN_POINT ( 'NONE',  ( 186.6899999999999977, 46.38749999999999574, -38.10000000000000142 ) ) ;
#38084=EDGE_CURVE ( 'NONE', #21668, #48266, #83798, .T. ) ;
#38214=AXIS2_PLACEMENT_3D ( 'NONE', #39503, #67202, #62176 ) ;
#38292=DIRECTION ( 'NONE',  ( 0.000000000000000000, 0.000000000000000000, 1.000000000000000000 ) ) ;
#38308=CARTESIAN_POINT ( 'NONE',  ( 173.9900000000000091, 68.61249999999999716, -35.28456447661465489 ) ) ;
#38348=ORIENTED_EDGE ( 'NONE', *, *, #2499, .T. ) ;
#38350=DIRECTION ( 'NONE',  ( -1.000000000000000000, 0.000000000000000000, 0.000000000000000000 ) ) ;
#38383=DIRECTION ( 'NONE',  ( -1.000000000000000000, 0.000000000000000000, 0.000000000000000000 ) ) ;
#38449=ORIENTED_EDGE ( 'NONE', *, *, #2499, .F. ) ;
#38455=VECTOR ( 'NONE', #30074, 1000.000000000000000 ) ;
#38498=AXIS2_PLACEMENT_3D ( 'NONE', #81824, #19138, #74996 ) ;
#38623=VERTEX_POINT ( 'NONE', #54521 ) ;
#38704=VECTOR ( 'NONE', #2157, 1000.000000000000000 ) ;
#38705=DIRECTION ( 'NONE',  ( 1.000000000000000000, 0.000000000000000000, 2.108231265501709878E-16 ) ) ;
#38723=DIRECTION ( 'NONE',  ( -0.7071067811865444641, 0.000000000000000000, 0.7071067811865505703 ) ) ;
#38861=DIRECTION ( 'NONE',  ( 0.000000000000000000, 0.000000000000000000, 1.000000000000000000 ) ) ;
#38862=ADVANCED_FACE ( 'NONE', ( #15916 ), #70430, .T. ) ;
#38918=CARTESIAN_POINT ( 'NONE',  ( 274.0659999999999741, 40.03750000000000142, -7.937500000000000000 ) ) ;
#38978=EDGE_LOOP ( 'NONE', ( #18033, #89718, #88007, #57496 ) ) ;
#38984=DIRECTION ( 'NONE',  ( -0.000000000000000000, 1.000000000000000000, 0.000000000000000000 ) ) ;
#39020=ORIENTED_EDGE ( 'NONE', *, *, #36104, .T. ) ;
#39057=CARTESIAN_POINT ( 'NONE',  ( 226.4410000000000025, 40.03750000000000142, -7.937500000000000000 ) ) ;
#39077=DIRECTION ( 'NONE',  ( 1.000000000000000000, 0.000000000000000000, 0.000000000000000000 ) ) ;
#39174=FACE_OUTER_BOUND ( 'NONE', #41253, .T. ) ;
#39209=CARTESIAN_POINT ( 'NONE',  ( 259.3340000000000032, 52.73749999999999716, 10.66800000000000104 ) ) ;
#39252=CARTESIAN_POINT ( 'NONE',  ( 248.6659999999999968, 52.73749999999999716, -2.903194600000015502 ) ) ;
#39503=CARTESIAN_POINT ( 'NONE',  ( 183.5150000000000148, 14.63749999999999929, -52.38749999999999574 ) ) ;
#39711=AXIS2_PLACEMENT_3D ( 'NONE', #29296, #19894, #61219 ) ;
#39779=CARTESIAN_POINT ( 'NONE',  ( 237.9979999999999905, 52.73749999999999716, 10.66800000000000104 ) ) ;
#39808=CARTESIAN_POINT ( 'NONE',  ( 186.6899999999999977, 59.08750000000000568, -38.10000000000000142 ) ) ;
#39836=EDGE_LOOP ( 'NONE', ( #65935, #28257, #40571, #48982 ) ) ;
#39840=PLANE ( 'NONE',  #2112 ) ;
#39872=FACE_OUTER_BOUND ( 'NONE', #13142, .T. ) ;
#39881=ORIENTED_EDGE ( 'NONE', *, *, #11437, .F. ) ;
#39899=ORIENTED_EDGE ( 'NONE', *, *, #12175, .T. ) ;
#39925=LINE ( 'NONE', #2407, #70686 ) ;
#39937=DIRECTION ( 'NONE',  ( 0.000000000000000000, 0.000000000000000000, 1.000000000000000000 ) ) ;
#39942=DIRECTION ( 'NONE',  ( -0.5000000000000003331, 0.8660254037844383745, 0.000000000000000000 ) ) ;
#39943=DIRECTION ( 'NONE',  ( 0.000000000000000000, 0.000000000000000000, 1.000000000000000000 ) ) ;
#39944=PLANE ( 'NONE',  #61105 ) ;
#40022=DIRECTION ( 'NONE',  ( 0.000000000000000000, 0.000000000000000000, -1.000000000000000000 ) ) ;
#40031=VECTOR ( 'NONE', #62091, 1000.000000000000114 ) ;
#40106=ORIENTED_EDGE ( 'NONE', *, *, #72238, .T. ) ;
#40123=DIRECTION ( 'NONE',  ( 1.000000000000000000, 0.000000000000000000, 0.000000000000000000 ) ) ;
#40140=LINE ( 'NONE', #67860, #78751 ) ;
#40155=DIRECTION ( 'NONE',  ( 0.000000000000000000, 1.000000000000000000, 0.000000000000000000 ) ) ;
#40156=CARTESIAN_POINT ( 'NONE',  ( 219.9639999999999986, 40.03750000000000142, -7.937500000000000000 ) ) ;
#40217=AXIS2_PLACEMENT_3D ( 'NONE', #59069, #78676, #17321 ) ;
#40249=CARTESIAN_POINT ( 'NONE',  ( 210.5660000000000025, 52.73749999999999716, -44.45000000000000284 ) ) ;
#40259=EDGE_CURVE ( 'NONE', #14890, #56634, #39925, .T. ) ;
#40266=AXIS2_PLACEMENT_3D ( 'NONE', #45247, #72539, #32075 ) ;
#40269=LINE ( 'NONE', #46626, #41932 ) ;
#40309=VECTOR ( 'NONE', #68620, 1000.000000000000000 ) ;
#40311=FACE_OUTER_BOUND ( 'NONE', #13416, .T. ) ;
#40315=VERTEX_POINT ( 'NONE', #46733 ) ;
#40322=AXIS2_PLACEMENT_3D ( 'NONE', #71332, #44037, #49959 ) ;
#40349=VECTOR ( 'NONE', #34945, 1000.000000000000000 ) ;
#40440=FACE_OUTER_BOUND ( 'NONE', #33614, .T. ) ;
#40554=VECTOR ( 'NONE', #78038, 1000.000000000000000 ) ;
#40571=ORIENTED_EDGE ( 'NONE', *, *, #12473, .T. ) ;
#40669=CIRCLE ( 'NONE', #14568, 9.810460662156732070 ) ;
#40707=CARTESIAN_POINT ( 'NONE',  ( 186.6899999999999977, 52.73749999999999716, -44.45000000000000284 ) ) ;
#40719=FACE_OUTER_BOUND ( 'NONE', #70777, .T. ) ;
#40723=AXIS2_PLACEMENT_3D ( 'NONE', #87741, #74555, #86413 ) ;
#40780=ORIENTED_EDGE ( 'NONE', *, *, #67005, .F. ) ;
#40793=EDGE_CURVE ( 'NONE', #64462, #11195, #27101, .T. ) ;
#40794=ORIENTED_EDGE ( 'NONE', *, *, #41066, .F. ) ;
#40844=CARTESIAN_POINT ( 'NONE',  ( 223.2659999999999911, 52.73749999999999716, -55.11800000000000210 ) ) ;
#41009=VECTOR ( 'NONE', #5493, 1000.000000000000000 ) ;
#41023=ORIENTED_EDGE ( 'NONE', *, *, #67005, .T. ) ;
#41066=EDGE_CURVE ( 'NONE', #54710, #59900, #59261, .T. ) ;
#41073=DIRECTION ( 'NONE',  ( 0.000000000000000000, 0.000000000000000000, -1.000000000000000000 ) ) ;
#41135=EDGE_CURVE ( 'NONE', #42703, #2727, #9795, .T. ) ;
#41166=EDGE_LOOP ( 'NONE', ( #72398, #62109, #28479, #57236 ) ) ;
#41189=LINE ( 'NONE', #68916, #40031 ) ;
#41200=CARTESIAN_POINT ( 'NONE',  ( 177.1649999999999920, 14.63749999999999929, -57.14999999999999858 ) ) ;
#41253=EDGE_LOOP ( 'NONE', ( #63944, #62652, #86211, #19360 ) ) ;
#41278=COLOUR_RGB ( '', 0.09019608, 0.27058824, 0.51372549) ;
#41284=CARTESIAN_POINT ( 'NONE',  ( 186.6899999999999977, 52.73749999999999716, -44.45000000000000284 ) ) ;
#41285=EDGE_CURVE ( 'NONE', #84828, #69678, #76029, .T. ) ;
#41367=AXIS2_PLACEMENT_3D ( 'NONE', #31129, #44756, #58828 ) ;
#41426=VECTOR ( 'NONE', #18179, 1000.000000000000000 ) ;
#41544=CARTESIAN_POINT ( 'NONE',  ( 255.9983484187079910, 65.43750000000000000, -2.032000000000000028 ) ) ;
#41574=LINE ( 'NONE', #76569, #77991 ) ;
#41575=AXIS2_PLACEMENT_3D ( 'NONE', #87722, #59104, #17347 ) ;
#41587=EDGE_CURVE ( 'NONE', #87914, #78380, #69062, .T. ) ;
#41610=EDGE_LOOP ( 'NONE', ( #55496, #9003, #25495, #72743 ) ) ;
#41650=ORIENTED_EDGE ( 'NONE', *, *, #59736, .T. ) ;
#41672=EDGE_LOOP ( 'NONE', ( #54527, #14504 ) ) ;
#41775=ORIENTED_EDGE ( 'NONE', *, *, #16373, .T. ) ;
#41786=FACE_OUTER_BOUND ( 'NONE', #71433, .T. ) ;
#41802=EDGE_CURVE ( 'NONE', #78558, #9584, #63535, .T. ) ;
#41823=CARTESIAN_POINT ( 'NONE',  ( 210.2301280605339855, 25.81350000000000477, -7.937500000000000000 ) ) ;
#41850=EDGE_CURVE ( 'NONE', #48266, #21668, #59233, .T. ) ;
#41852=PLANE ( 'NONE',  #69572 ) ;
#41932=VECTOR ( 'NONE', #7112, 1000.000000000000000 ) ;
#41957=CYLINDRICAL_SURFACE ( 'NONE', #72978, 12.44599999999999795 ) ;
#41992=ORIENTED_EDGE ( 'NONE', *, *, #21263, .F. ) ;
#42058=DIRECTION ( 'NONE',  ( -0.7071067811865470176, -0.7071067811865480168, 0.000000000000000000 ) ) ;
#42075=EDGE_CURVE ( 'NONE', #44015, #30543, #26117, .T. ) ;
#42088=VECTOR ( 'NONE', #20133, 1000.000000000000114 ) ;
#42196=ORIENTED_EDGE ( 'NONE', *, *, #18201, .T. ) ;
#42233=DIRECTION ( 'NONE',  ( 0.4999999999999998890, 0.8660254037844387076, 0.000000000000000000 ) ) ;
#42260=VECTOR ( 'NONE', #37531, 1000.000000000000114 ) ;
#42322=VECTOR ( 'NONE', #64632, 1000.000000000000000 ) ;
#42451=VERTEX_POINT ( 'NONE', #45968 ) ;
#42499=DIRECTION ( 'NONE',  ( 1.000000000000000000, 0.000000000000000000, 2.108231265501709878E-16 ) ) ;
#42510=DIRECTION ( 'NONE',  ( -1.000000000000000000, 0.000000000000000000, -2.108231265501709878E-16 ) ) ;
#42645=ORIENTED_EDGE ( 'NONE', *, *, #82969, .T. ) ;
#42680=DIRECTION ( 'NONE',  ( -1.000000000000000000, 0.000000000000000000, 0.000000000000000000 ) ) ;
#42703=VERTEX_POINT ( 'NONE', #15066 ) ;
#42837=AXIS2_PLACEMENT_3D ( 'NONE', #25630, #78838, #16597 ) ;
#42864=CARTESIAN_POINT ( 'NONE',  ( 239.7378999999999962, 52.73749999999999716, -2.903194600000015502 ) ) ;
#42882=AXIS2_PLACEMENT_3D ( 'NONE', #41823, #75481, #44515 ) ;
#42961=CARTESIAN_POINT ( 'NONE',  ( 245.4909999999999854, 40.03750000000000142, -67.11950000000000216 ) ) ;
#42989=VERTEX_POINT ( 'NONE', #63904 ) ;
#43091=EDGE_CURVE ( 'NONE', #55699, #26649, #52454, .T. ) ;
#43292=EDGE_LOOP ( 'NONE', ( #29517, #62201, #35355, #73500 ) ) ;
#43310=AXIS2_PLACEMENT_3D ( 'NONE', #75527, #14191, #69608 ) ;
#43380=CARTESIAN_POINT ( 'NONE',  ( 183.5150000000000148, 14.63749999999999929, -14.28749999999999964 ) ) ;
#43399=LINE ( 'NONE', #21189, #65166 ) ;
#43408=CARTESIAN_POINT ( 'NONE',  ( 186.6899999999999977, 46.38749999999999574, -50.79999999999999716 ) ) ;
#43429=EDGE_CURVE ( 'NONE', #22107, #2953, #73837, .T. ) ;
#43468=LINE ( 'NONE', #58882, #20634 ) ;
#43478=CARTESIAN_POINT ( 'NONE',  ( 263.3306968374159851, 52.73749999999999716, 10.66800000000000104 ) ) ;
#43491=ORIENTED_EDGE ( 'NONE', *, *, #64168, .F. ) ;
#43643=LINE ( 'NONE', #29579, #88170 ) ;
#43678=ORIENTED_EDGE ( 'NONE', *, *, #77090, .T. ) ;
#43822=ORIENTED_EDGE ( 'NONE', *, *, #49052, .F. ) ;
#43892=DIRECTION ( 'NONE',  ( 0.000000000000000000, 0.000000000000000000, 1.000000000000000000 ) ) ;
#43952=EDGE_LOOP ( 'NONE', ( #65877, #14478 ) ) ;
#44015=VERTEX_POINT ( 'NONE', #58195 ) ;
#44037=DIRECTION ( 'NONE',  ( 0.8660254037844384856, 0.5000000000000003331, 0.000000000000000000 ) ) ;
#44147=FACE_OUTER_BOUND ( 'NONE', #88364, .T. ) ;
#44158=( NAMED_UNIT ( * ) SI_UNIT ( $, .STERADIAN. ) SOLID_ANGLE_UNIT ( ) );
#44170=EDGE_CURVE ( 'NONE', #87657, #32855, #17755, .T. ) ;
#44189=CARTESIAN_POINT ( 'NONE',  ( 173.9900000000000091, 5.112500000000000711, -7.937500000000000000 ) ) ;
#44206=DIRECTION ( 'NONE',  ( -0.000000000000000000, -0.000000000000000000, -1.000000000000000000 ) ) ;
#44209=ORIENTED_EDGE ( 'NONE', *, *, #62430, .F. ) ;
#44214=CARTESIAN_POINT ( 'NONE',  ( 70.98999999999998067, 52.73749999999999716, -52.28750000000002274 ) ) ;
#44288=CARTESIAN_POINT ( 'NONE',  ( 183.5150000000000148, 14.63749999999999929, -14.28749999999999964 ) ) ;
#44317=CARTESIAN_POINT ( 'NONE',  ( 177.1649999999999920, 14.63749999999999929, -52.38749999999999574 ) ) ;
#44319=LINE ( 'NONE', #65230, #11306 ) ;
#44326=DIRECTION ( 'NONE',  ( -1.000000000000000000, 0.000000000000000000, 7.136255983449500255E-16 ) ) ;
#44328=CARTESIAN_POINT ( 'NONE',  ( 226.4410000000000025, 40.03750000000000142, -63.94449999999999790 ) ) ;
#44408=VECTOR ( 'NONE', #87372, 999.9999999999998863 ) ;
#44515=DIRECTION ( 'NONE',  ( 0.000000000000000000, 0.000000000000000000, 1.000000000000000000 ) ) ;
#44676=ORIENTED_EDGE ( 'NONE', *, *, #40793, .T. ) ;
#44682=LINE ( 'NONE', #2482, #65243 ) ;
#44756=DIRECTION ( 'NONE',  ( 0.000000000000000000, 0.000000000000000000, 1.000000000000000000 ) ) ;
#44770=DIRECTION ( 'NONE',  ( -1.000000000000000000, 0.000000000000000000, 0.000000000000000000 ) ) ;
#44788=ORIENTED_EDGE ( 'NONE', *, *, #14206, .F. ) ;
#44824=CARTESIAN_POINT ( 'NONE',  ( 199.3900000000000148, 46.38749999999999574, -38.10000000000000142 ) ) ;
#44847=VECTOR ( 'NONE', #66558, 1000.000000000000000 ) ;
#44852=ADVANCED_FACE ( 'NONE', ( #70159 ), #14590, .T. ) ;
#44864=CARTESIAN_POINT ( 'NONE',  ( 173.9900000000000091, 14.32000000000000028, -71.37400000000000944 ) ) ;
#44911=ORIENTED_EDGE ( 'NONE', *, *, #37983, .F. ) ;
#44915=DIRECTION ( 'NONE',  ( 1.000000000000000000, 0.000000000000000000, 2.108231265501709878E-16 ) ) ;
#44945=EDGE_LOOP ( 'NONE', ( #21665, #24078, #27120, #33554 ) ) ;
#44988=AXIS2_PLACEMENT_3D ( 'NONE', #87515, #25276, #52942 ) ;
#44989=LINE ( 'NONE', #50470, #67577 ) ;
#45024=CARTESIAN_POINT ( 'NONE',  ( 177.1649999999999920, 25.81350000000000477, -7.937500000000000000 ) ) ;
#45056=DIRECTION ( 'NONE',  ( 0.000000000000000000, 0.000000000000000000, -1.000000000000000000 ) ) ;
#45130=ORIENTED_EDGE ( 'NONE', *, *, #3471, .F. ) ;
#45144=LINE ( 'NONE', #25610, #14874 ) ;
#45154=LINE ( 'NONE', #17907, #687 ) ;
#45164=CARTESIAN_POINT ( 'NONE',  ( 213.4642805167760002, 52.73749999999999716, -34.63953933784325301 ) ) ;
#45171=ORIENTED_EDGE ( 'NONE', *, *, #73227, .F. ) ;
#45177=CARTESIAN_POINT ( 'NONE',  ( 186.6899999999999977, 46.38749999999999574, -50.79999999999999716 ) ) ;
#45247=CARTESIAN_POINT ( 'NONE',  ( 204.2160000000000082, 52.73749999999999716, -44.45000000000000284 ) ) ;
#45481=CARTESIAN_POINT ( 'NONE',  ( 183.5150000000000148, 52.73749999999999716, -44.45000000000000284 ) ) ;
#45521=PLANE ( 'NONE',  #50053 ) ;
#45591=DIRECTION ( 'NONE',  ( -1.000000000000000000, 0.000000000000000000, 0.000000000000000000 ) ) ;
#45615=AXIS2_PLACEMENT_3D ( 'NONE', #45710, #59797, #30774 ) ;
#45626=CARTESIAN_POINT ( 'NONE',  ( 257.5940999999999690, 52.73749999999999716, -2.903194600000015502 ) ) ;
#45655=AXIS2_PLACEMENT_3D ( 'NONE', #10645, #38350, #32417 ) ;
#45662=FACE_OUTER_BOUND ( 'NONE', #19857, .T. ) ;
#45685=CARTESIAN_POINT ( 'NONE',  ( 274.0659999999999741, 36.86249999999999716, -58.73749999999999716 ) ) ;
#45710=CARTESIAN_POINT ( 'NONE',  ( 235.9910211978967141, -11.20588573913161134, -10.97647784993501396 ) ) ;
#45755=ORIENTED_EDGE ( 'NONE', *, *, #40793, .F. ) ;
#45786=ORIENTED_EDGE ( 'NONE', *, *, #21202, .F. ) ;
#45795=CARTESIAN_POINT ( 'NONE',  ( 186.6899999999999977, 46.38749999999999574, -38.10000000000000142 ) ) ;
#45817=CARTESIAN_POINT ( 'NONE',  ( 234.0013031625829854, 52.73749999999999716, -2.032000000000000028 ) ) ;
#45846=AXIS2_PLACEMENT_3D ( 'NONE', #67565, #80761, #33041 ) ;
#45862=DIRECTION ( 'NONE',  ( 0.000000000000000000, 0.000000000000000000, -1.000000000000000000 ) ) ;
#45963=CARTESIAN_POINT ( 'NONE',  ( 226.4410000000000025, 65.43750000000000000, -63.94449999999999790 ) ) ;
#45968=CARTESIAN_POINT ( 'NONE',  ( 226.4410000000000025, 65.43750000000000000, -63.94449999999999790 ) ) ;
#45978=EDGE_CURVE ( 'NONE', #28622, #13566, #4972, .T. ) ;
#45990=ORIENTED_EDGE ( 'NONE', *, *, #84936, .T. ) ;
#46078=EDGE_CURVE ( 'NONE', #12759, #25005, #14024, .T. ) ;
#46147=EDGE_CURVE ( 'NONE', #71852, #82635, #49562, .T. ) ;
#46218=ORIENTED_EDGE ( 'NONE', *, *, #58185, .T. ) ;
#46263=EDGE_LOOP ( 'NONE', ( #76998, #3760 ) ) ;
#46298=FACE_OUTER_BOUND ( 'NONE', #83895, .T. ) ;
#46304=VERTEX_POINT ( 'NONE', #15385 ) ;
#46312=ORIENTED_EDGE ( 'NONE', *, *, #12325, .F. ) ;
#46339=CIRCLE ( 'NONE', #18804, 10.66800000000000992 ) ;
#46350=CARTESIAN_POINT ( 'NONE',  ( 177.1649999999999920, 14.63749999999999929, -14.28749999999999964 ) ) ;
#46409=ORIENTED_EDGE ( 'NONE', *, *, #6491, .F. ) ;
#46487=DIRECTION ( 'NONE',  ( -1.000000000000000000, 0.000000000000000000, -2.108231265501709878E-16 ) ) ;
#46538=ORIENTED_EDGE ( 'NONE', *, *, #89339, .F. ) ;
#46576=VECTOR ( 'NONE', #44915, 1000.000000000000000 ) ;
#46626=CARTESIAN_POINT ( 'NONE',  ( 173.9900000000000091, 68.61249999999999716, -53.61543552338530105 ) ) ;
#46733=CARTESIAN_POINT ( 'NONE',  ( 173.9900000000000091, 5.112500000000000711, -58.73749999999999716 ) ) ;
#46826=PLANE ( 'NONE',  #40723 ) ;
#46875=CARTESIAN_POINT ( 'NONE',  ( 255.9983484187079910, 65.43750000000000000, -2.032000000000000028 ) ) ;
#46894=DIRECTION ( 'NONE',  ( -7.136255983449500255E-16, 0.000000000000000000, -1.000000000000000000 ) ) ;
#46926=DIRECTION ( 'NONE',  ( 1.000000000000000000, 0.000000000000000000, 0.000000000000000000 ) ) ;
#47032=VERTEX_POINT ( 'NONE', #51549 ) ;
#47034=ORIENTED_EDGE ( 'NONE', *, *, #86010, .F. ) ;
#47067=CARTESIAN_POINT ( 'NONE',  ( 274.0659999999999741, 40.03750000000000142, -7.937500000000000000 ) ) ;
#47178=DIRECTION ( 'NONE',  ( 1.000000000000000000, 0.000000000000000000, 0.000000000000000000 ) ) ;
#47225=VERTEX_POINT ( 'NONE', #82154 ) ;
#47290=SHAPE_REPRESENTATION ( 'Proximity Switch Housing', ( #50656 ), #7165 ) ;
#47307=EDGE_LOOP ( 'NONE', ( #31249, #1756 ) ) ;
#47313=CARTESIAN_POINT ( 'NONE',  ( 242.3160000000000025, 40.03750000000000142, -63.94449999999999790 ) ) ;
#47326=DIRECTION ( 'NONE',  ( 1.000000000000000000, -2.098553464303459752E-16, 0.000000000000000000 ) ) ;
#47449=CARTESIAN_POINT ( 'NONE',  ( 199.3900000000000148, 46.38749999999999574, -38.10000000000000142 ) ) ;
#47477=VERTEX_POINT ( 'NONE', #49380 ) ;
#47504=LINE ( 'NONE', #26630, #69855 ) ;
#47539=CIRCLE ( 'NONE', #69350, 4.762500000000001066 ) ;
#47540=CARTESIAN_POINT ( 'NONE',  ( 173.9900000000000091, 28.98850000000000193, -7.937500000000000000 ) ) ;
#47549=DIRECTION ( 'NONE',  ( 0.000000000000000000, 5.463695987328529395E-16, -1.000000000000000000 ) ) ;
#47564=CARTESIAN_POINT ( 'NONE',  ( 213.7409999999999854, 52.73749999999999716, -44.45000000000000284 ) ) ;
#47630=AXIS2_PLACEMENT_3D ( 'NONE', #50395, #30418, #78140 ) ;
#47644=CARTESIAN_POINT ( 'NONE',  ( 213.7409999999999854, 52.73749999999999716, -51.09754249571540186 ) ) ;
#47647=AXIS2_PLACEMENT_3D ( 'NONE', #65967, #60039, #17830 ) ;
#47648=VECTOR ( 'NONE', #113, 1000.000000000000000 ) ;
#47681=LINE ( 'NONE', #75416, #57593 ) ;
#47728=EDGE_LOOP ( 'NONE', ( #33576, #66242 ) ) ;
#47775=LINE ( 'NONE', #34152, #69012 ) ;
#47777=CARTESIAN_POINT ( 'NONE',  ( 248.6659999999999968, 52.73749999999999716, -2.903194600000015502 ) ) ;
#47808=CARTESIAN_POINT ( 'NONE',  ( 241.3336515812914911, 65.43750000000000000, -2.032000000000000028 ) ) ;
#47814=ORIENTED_EDGE ( 'NONE', *, *, #67623, .F. ) ;
#48006=ADVANCED_FACE ( 'NONE', ( #88012 ), #39840, .T. ) ;
#48008=LINE ( 'NONE', #54816, #6437 ) ;
#48085=CIRCLE ( 'NONE', #84381, 3.174999999999997158 ) ;
#48137=EDGE_LOOP ( 'NONE', ( #46312, #36148, #34747, #84846 ) ) ;
#48169=LINE ( 'NONE', #69987, #28122 ) ;
#48222=EDGE_CURVE ( 'NONE', #55564, #83557, #34113, .T. ) ;
#48265=LINE ( 'NONE', #21495, #77240 ) ;
#48266=VERTEX_POINT ( 'NONE', #7583 ) ;
#48331=ORIENTED_EDGE ( 'NONE', *, *, #12473, .F. ) ;
#48336=DIRECTION ( 'NONE',  ( 0.000000000000000000, 5.463695987328529395E-16, -1.000000000000000000 ) ) ;
#48352=CARTESIAN_POINT ( 'NONE',  ( 248.6659999999999968, 52.73749999999999716, 10.66800000000000104 ) ) ;
#48452=ADVANCED_FACE ( 'NONE', ( #80652 ), #85690, .T. ) ;
#48582=CONICAL_SURFACE ( 'NONE', #71831, 10.66799999999999748, 0.08726646259971625186 ) ;
#48617=VECTOR ( 'NONE', #8474, 1000.000000000000000 ) ;
#48715=DIRECTION ( 'NONE',  ( 0.000000000000000000, -1.000000000000000000, 0.000000000000000000 ) ) ;
#48822=DIRECTION ( 'NONE',  ( 1.000000000000000000, 0.000000000000000000, 0.000000000000000000 ) ) ;
#48827=ORIENTED_EDGE ( 'NONE', *, *, #40259, .T. ) ;
#48845=ORIENTED_EDGE ( 'NONE', *, *, #67538, .T. ) ;
#48898=DIRECTION ( 'NONE',  ( 1.000000000000000000, 0.000000000000000000, 0.000000000000000000 ) ) ;
#48982=ORIENTED_EDGE ( 'NONE', *, *, #36381, .F. ) ;
#48990=LINE ( 'NONE', #21317, #82129 ) ;
#49052=EDGE_CURVE ( 'NONE', #16389, #64803, #47775, .T. ) ;
#49065=EDGE_CURVE ( 'NONE', #30543, #78177, #60512, .T. ) ;
#49119=CARTESIAN_POINT ( 'NONE',  ( 210.5660000000000025, 52.73749999999999716, -44.45000000000000284 ) ) ;
#49207=ORIENTED_EDGE ( 'NONE', *, *, #49557, .F. ) ;
#49231=DIRECTION ( 'NONE',  ( 1.000000000000000000, 0.000000000000000000, 0.000000000000000000 ) ) ;
#49259=ORIENTED_EDGE ( 'NONE', *, *, #31531, .F. ) ;
#49281=FACE_OUTER_BOUND ( 'NONE', #58107, .T. ) ;
#49365=ORIENTED_EDGE ( 'NONE', *, *, #57784, .F. ) ;
#49373=AXIS2_PLACEMENT_3D ( 'NONE', #71076, #57418, #8850 ) ;
#49380=CARTESIAN_POINT ( 'NONE',  ( 177.1649999999999920, 5.112500000000000711, -7.937500000000000000 ) ) ;
#49423=EDGE_CURVE ( 'NONE', #60085, #14890, #44989, .T. ) ;
#49449=VECTOR ( 'NONE', #49687, 1000.000000000000000 ) ;
#49492=LINE ( 'NONE', #55846, #17281 ) ;
#49557=EDGE_CURVE ( 'NONE', #13223, #16389, #80429, .T. ) ;
#49562=CIRCLE ( 'NONE', #20601, 4.762500000000002842 ) ;
#49588=VECTOR ( 'NONE', #58009, 1000.000000000000000 ) ;
#49599=VECTOR ( 'NONE', #87755, 1000.000000000000000 ) ;
#49611=ORIENTED_EDGE ( 'NONE', *, *, #27620, .T. ) ;
#49646=ORIENTED_EDGE ( 'NONE', *, *, #59807, .T. ) ;
#49660=ORIENTED_EDGE ( 'NONE', *, *, #66395, .T. ) ;
#49674=DIRECTION ( 'NONE',  ( 1.000000000000000000, 0.000000000000000000, 0.000000000000000000 ) ) ;
#49687=DIRECTION ( 'NONE',  ( -1.000000000000000000, 0.000000000000000000, -2.108231265501709878E-16 ) ) ;
#49748=FACE_OUTER_BOUND ( 'NONE', #81040, .T. ) ;
#49759=CARTESIAN_POINT ( 'NONE',  ( 183.5150000000000148, 68.61249999999999716, -35.28456447661459805 ) ) ;
#49770=CIRCLE ( 'NONE', #74481, 9.524999999999998579 ) ;
#49808=ADVANCED_FACE ( 'NONE', ( #86138 ), #87915, .F. ) ;
#49817=ORIENTED_EDGE ( 'NONE', *, *, #78101, .T. ) ;
#49843=ADVANCED_FACE ( 'NONE', ( #74733 ), #81572, .T. ) ;
#49905=CARTESIAN_POINT ( 'NONE',  ( 255.9983484187079910, 40.03750000000000142, -2.032000000000000028 ) ) ;
#49959=DIRECTION ( 'NONE',  ( 0.000000000000000000, 0.000000000000000000, -1.000000000000000000 ) ) ;
#49984=EDGE_CURVE ( 'NONE', #26649, #17992, #54248, .T. ) ;
#50020=FACE_OUTER_BOUND ( 'NONE', #34912, .T. ) ;
#50053=AXIS2_PLACEMENT_3D ( 'NONE', #60503, #87343, #66882 ) ;
#50129=AXIS2_PLACEMENT_3D ( 'NONE', #69963, #34976, #917 ) ;
#50209=CARTESIAN_POINT ( 'NONE',  ( 219.9639999999999986, 40.03750000000000142, -7.937500000000000000 ) ) ;
#50220=ORIENTED_EDGE ( 'NONE', *, *, #49423, .T. ) ;
#50342=ORIENTED_EDGE ( 'NONE', *, *, #85503, .F. ) ;
#50369=DIRECTION ( 'NONE',  ( 0.000000000000000000, 0.000000000000000000, -1.000000000000000000 ) ) ;
#50378=ORIENTED_EDGE ( 'NONE', *, *, #75148, .F. ) ;
#50383=CARTESIAN_POINT ( 'NONE',  ( 173.9900000000000091, 68.61249999999999716, -35.28456447661459805 ) ) ;
#50384=VECTOR ( 'NONE', #54709, 1000.000000000000000 ) ;
#50395=CARTESIAN_POINT ( 'NONE',  ( 213.7409999999999854, 52.73749999999999716, -37.80245750428454699 ) ) ;
#50423=DIRECTION ( 'NONE',  ( -1.000000000000000000, 0.000000000000000000, 0.000000000000000000 ) ) ;
#50444=DIRECTION ( 'NONE',  ( 0.000000000000000000, 0.000000000000000000, 1.000000000000000000 ) ) ;
#50470=CARTESIAN_POINT ( 'NONE',  ( 219.9639999999999986, 40.03750000000000142, -7.937500000000000000 ) ) ;
#50473=CARTESIAN_POINT ( 'NONE',  ( 274.0659999999999741, 36.86249999999999716, -7.937500000000000000 ) ) ;
#50626=EDGE_CURVE ( 'NONE', #76956, #4611, #47681, .T. ) ;
#50656=AXIS2_PLACEMENT_3D ( 'NONE', #89656, #19265, #5642 ) ;
#50773=ORIENTED_EDGE ( 'NONE', *, *, #64643, .F. ) ;
#50791=PLANE ( 'NONE',  #83047 ) ;
#50798=EDGE_CURVE ( 'NONE', #59868, #6360, #84488, .T. ) ;
#50838=CARTESIAN_POINT ( 'NONE',  ( 226.4410000000000025, 65.43750000000000000, -2.032000000000000028 ) ) ;
#50862=DIRECTION ( 'NONE',  ( -1.000000000000000000, 0.000000000000000000, 0.000000000000000000 ) ) ;
#50907=ORIENTED_EDGE ( 'NONE', *, *, #49984, .F. ) ;
#50908=EDGE_CURVE ( 'NONE', #42989, #78177, #2696, .T. ) ;
#50926=DIRECTION ( 'NONE',  ( 1.000000000000000000, 0.000000000000000000, 0.000000000000000000 ) ) ;
#50960=AXIS2_PLACEMENT_3D ( 'NONE', #49759, #70675, #76592 ) ;
#50977=DIRECTION ( 'NONE',  ( 0.000000000000000000, 0.000000000000000000, -1.000000000000000000 ) ) ;
#50986=CARTESIAN_POINT ( 'NONE',  ( 173.9900000000000091, 36.86249999999999716, -53.61543552338530105 ) ) ;
#50988=CARTESIAN_POINT ( 'NONE',  ( 213.4642805167760002, 52.73749999999999716, -44.45000000000000284 ) ) ;
#51080=ORIENTED_EDGE ( 'NONE', *, *, #38084, .F. ) ;
#51390=CARTESIAN_POINT ( 'NONE',  ( 183.5150000000000148, 14.63749999999999929, -14.28749999999999964 ) ) ;
#51482=AXIS2_PLACEMENT_3D ( 'NONE', #18398, #73820, #37077 ) ;
#51486=ORIENTED_EDGE ( 'NONE', *, *, #76098, .T. ) ;
#51490=DIRECTION ( 'NONE',  ( -1.000000000000000000, 0.000000000000000000, -2.108231265501709878E-16 ) ) ;
#51549=CARTESIAN_POINT ( 'NONE',  ( 223.2659999999999911, 52.73749999999999716, -33.78199999999999648 ) ) ;
#51582=VECTOR ( 'NONE', #4815, 1000.000000000000000 ) ;
#51585=DIRECTION ( 'NONE',  ( 0.000000000000000000, 1.000000000000000000, 0.000000000000000000 ) ) ;
#51631=ORIENTED_EDGE ( 'NONE', *, *, #23264, .F. ) ;
#51632=LINE ( 'NONE', #79377, #25767 ) ;
#51633=PLANE ( 'NONE',  #44988 ) ;
#51668=FACE_BOUND ( 'NONE', #32843, .T. ) ;
#51696=CARTESIAN_POINT ( 'NONE',  ( 186.6899999999999977, 59.08750000000000568, -50.79999999999999716 ) ) ;
#51818=ORIENTED_EDGE ( 'NONE', *, *, #59807, .F. ) ;
#51969=CARTESIAN_POINT ( 'NONE',  ( 226.4410000000000025, 40.03750000000000142, -63.94449999999999790 ) ) ;
#51976=AXIS2_PLACEMENT_3D ( 'NONE', #40249, #60687, #33443 ) ;
#52072=CARTESIAN_POINT ( 'NONE',  ( 70.98999999999998067, 52.73749999999999716, -44.45000000000002416 ) ) ;
#52105=ORIENTED_EDGE ( 'NONE', *, *, #17799, .F. ) ;
#52186=DIRECTION ( 'NONE',  ( -1.000000000000000000, 0.000000000000000000, 0.000000000000000000 ) ) ;
#52226=CARTESIAN_POINT ( 'NONE',  ( 208.9149999999999920, 28.98850000000000193, -7.937500000000000000 ) ) ;
#52250=DIRECTION ( 'NONE',  ( 0.000000000000000000, 0.000000000000000000, 1.000000000000000000 ) ) ;
#52278=ORIENTED_EDGE ( 'NONE', *, *, #1006, .T. ) ;
#52408=ADVANCED_FACE ( 'NONE', ( #19388 ), #73903, .T. ) ;
#52454=LINE ( 'NONE', #17961, #44847 ) ;
#52473=ORIENTED_EDGE ( 'NONE', *, *, #58850, .F. ) ;
#52478=CARTESIAN_POINT ( 'NONE',  ( 274.0659999999999741, 36.86249999999999716, -7.937500000000000000 ) ) ;
#52567=ADVANCED_FACE ( 'NONE', ( #27100 ), #13920, .F. ) ;
#52576=VECTOR ( 'NONE', #2439, 1000.000000000000000 ) ;
#52589=VECTOR ( 'NONE', #59084, 1000.000000000000000 ) ;
#52617=VECTOR ( 'NONE', #80345, 1000.000000000000000 ) ;
#52637=ORIENTED_EDGE ( 'NONE', *, *, #64643, .T. ) ;
#52699=AXIS2_PLACEMENT_3D ( 'NONE', #44317, #37529, #72047 ) ;
#52702=DIRECTION ( 'NONE',  ( 1.000000000000000000, 0.000000000000000000, 0.000000000000000000 ) ) ;
#52729=DIRECTION ( 'NONE',  ( 1.000000000000000000, 0.000000000000000000, 0.000000000000000000 ) ) ;
#52747=DIRECTION ( 'NONE',  ( 0.000000000000000000, 0.000000000000000000, 1.000000000000000000 ) ) ;
#52770=ADVANCED_FACE ( 'NONE', ( #77949 ), #86549, .F. ) ;
#52777=EDGE_CURVE ( 'NONE', #54390, #42703, #1649, .T. ) ;
#52784=VERTEX_POINT ( 'NONE', #71137 ) ;
#52789=ORIENTED_EDGE ( 'NONE', *, *, #77880, .F. ) ;
#52803=LINE ( 'NONE', #18328, #16130 ) ;
#52824=DIRECTION ( 'NONE',  ( 0.000000000000000000, 1.000000000000000000, 0.000000000000000000 ) ) ;
#52847=ORIENTED_EDGE ( 'NONE', *, *, #85741, .T. ) ;
#52859=AXIS2_PLACEMENT_3D ( 'NONE', #28522, #14922, #35788 ) ;
#52875=CIRCLE ( 'NONE', #55742, 10.66800000000000992 ) ;
#52912=( GEOMETRIC_REPRESENTATION_CONTEXT ( 3 ) GLOBAL_UNCERTAINTY_ASSIGNED_CONTEXT ( ( #30550 ) ) GLOBAL_UNIT_ASSIGNED_CONTEXT ( ( #31626, #10732, #24386 ) ) REPRESENTATION_CONTEXT ( 'NONE', 'WORKASPACE' ) );
#52942=DIRECTION ( 'NONE',  ( 1.000000000000000000, 0.000000000000000000, 0.000000000000000000 ) ) ;
#53063=FACE_OUTER_BOUND ( 'NONE', #57132, .T. ) ;
#53092=DIRECTION ( 'NONE',  ( 0.000000000000000000, 1.000000000000000000, 0.000000000000000000 ) ) ;
#53095=DIRECTION ( 'NONE',  ( 0.000000000000000000, 0.000000000000000000, 1.000000000000000000 ) ) ;
#53138=LINE ( 'NONE', #58638, #65944 ) ;
#53165=EDGE_LOOP ( 'NONE', ( #32874, #39899, #48827, #59638, #44209, #61823 ) ) ;
#53236=FACE_OUTER_BOUND ( 'NONE', #24590, .T. ) ;
#53283=DIRECTION ( 'NONE',  ( 0.000000000000000000, 0.8660254037844387076, 0.4999999999999998890 ) ) ;
#53284=FACE_BOUND ( 'NONE', #41672, .T. ) ;
#53415=PLANE ( 'NONE',  #45615 ) ;
#53450=EDGE_CURVE ( 'NONE', #52784, #2982, #4821, .T. ) ;
#53501=ORIENTED_EDGE ( 'NONE', *, *, #4941, .T. ) ;
#53567=ORIENTED_EDGE ( 'NONE', *, *, #55400, .F. ) ;
#53611=ORIENTED_EDGE ( 'NONE', *, *, #30720, .F. ) ;
#53679=ORIENTED_EDGE ( 'NONE', *, *, #87208, .T. ) ;
#53707=EDGE_LOOP ( 'NONE', ( #21859, #20244, #36270, #67705 ) ) ;
#53798=CIRCLE ( 'NONE', #13179, 7.837499999999996803 ) ;
#53840=ORIENTED_EDGE ( 'NONE', *, *, #30986, .F. ) ;
#53855=CARTESIAN_POINT ( 'NONE',  ( 199.3900000000000148, 59.08750000000000568, -38.10000000000000142 ) ) ;
#53916=AXIS2_PLACEMENT_3D ( 'NONE', #85992, #39937, #33133 ) ;
#53921=VECTOR ( 'NONE', #33553, 1000.000000000000000 ) ;
#53942=EDGE_LOOP ( 'NONE', ( #7203, #73452, #29072, #34110 ) ) ;
#53970=LINE ( 'NONE', #6744, #53921 ) ;
#54000=CARTESIAN_POINT ( 'NONE',  ( 177.1649999999999920, 5.112500000000000711, -7.937500000000000000 ) ) ;
#54011=CARTESIAN_POINT ( 'NONE',  ( 210.5660000000000025, 52.73749999999999716, -39.68750000000000000 ) ) ;
#54013=PLANE ( 'NONE',  #76267 ) ;
#54077=DIRECTION ( 'NONE',  ( 0.8660254037844387076, -0.4999999999999998890, 0.000000000000000000 ) ) ;
#54108=DIRECTION ( 'NONE',  ( 0.000000000000000000, -1.000000000000000000, 0.000000000000000000 ) ) ;
#54111=AXIS2_PLACEMENT_3D ( 'NONE', #36897, #29197, #7843 ) ;
#54135=CIRCLE ( 'NONE', #58505, 10.66799999999999748 ) ;
#54248=LINE ( 'NONE', #47449, #3838 ) ;
#54266=VERTEX_POINT ( 'NONE', #87893 ) ;
#54322=PLANE ( 'NONE',  #54388 ) ;
#54326=AXIS2_PLACEMENT_3D ( 'NONE', #59526, #24584, #10944 ) ;
#54388=AXIS2_PLACEMENT_3D ( 'NONE', #47067, #33462, #82092 ) ;
#54390=VERTEX_POINT ( 'NONE', #76948 ) ;
#54415=EDGE_LOOP ( 'NONE', ( #80689, #11779 ) ) ;
#54416=CYLINDRICAL_SURFACE ( 'NONE', #275, 7.837499999999996803 ) ;
#54417=VERTEX_POINT ( 'NONE', #61507 ) ;
#54521=CARTESIAN_POINT ( 'NONE',  ( 219.9639999999999986, 40.03750000000000142, -58.73749999999999716 ) ) ;
#54527=ORIENTED_EDGE ( 'NONE', *, *, #59736, .F. ) ;
#54541=EDGE_CURVE ( 'NONE', #25005, #47477, #71924, .T. ) ;
#54659=VECTOR ( 'NONE', #28172, 1000.000000000000000 ) ;
#54664=VECTOR ( 'NONE', #32521, 1000.000000000000000 ) ;
#54672=VERTEX_POINT ( 'NONE', #12369 ) ;
#54691=ADVANCED_FACE ( 'NONE', ( #39174 ), #60961, .F. ) ;
#54709=DIRECTION ( 'NONE',  ( 0.000000000000000000, 0.000000000000000000, 1.000000000000000000 ) ) ;
#54710=VERTEX_POINT ( 'NONE', #32802 ) ;
#54769=CARTESIAN_POINT ( 'NONE',  ( 242.3160000000000025, 65.43750000000000000, -63.94449999999999790 ) ) ;
#54770=DIRECTION ( 'NONE',  ( -1.000000000000000000, 0.000000000000000000, -2.108231265501709878E-16 ) ) ;
#54782=VERTEX_POINT ( 'NONE', #87778 ) ;
#54791=EDGE_CURVE ( 'NONE', #47032, #84299, #54135, .T. ) ;
#54801=CARTESIAN_POINT ( 'NONE',  ( 186.6899999999999977, 46.38749999999999574, -38.10000000000000142 ) ) ;
#54805=EDGE_CURVE ( 'NONE', #31184, #78791, #82777, .T. ) ;
#54816=CARTESIAN_POINT ( 'NONE',  ( 183.5150000000000148, 14.63749999999999929, -57.14999999999999858 ) ) ;
#54953=CYLINDRICAL_SURFACE ( 'NONE', #6476, 4.762500000000002842 ) ;
#54970=ORIENTED_EDGE ( 'NONE', *, *, #10817, .F. ) ;
#55015=AXIS2_PLACEMENT_3D ( 'NONE', #73668, #11451, #32320 ) ;
#55048=VECTOR ( 'NONE', #38723, 1000.000000000000114 ) ;
#55231=ORIENTED_EDGE ( 'NONE', *, *, #76098, .F. ) ;
#55244=DIRECTION ( 'NONE',  ( 1.000000000000000000, 0.000000000000000000, 0.000000000000000000 ) ) ;
#55333=EDGE_CURVE ( 'NONE', #84665, #40315, #83438, .T. ) ;
#55338=EDGE_LOOP ( 'NONE', ( #22247, #3128 ) ) ;
#55358=DIRECTION ( 'NONE',  ( 0.000000000000000000, 0.000000000000000000, -1.000000000000000000 ) ) ;
#55400=EDGE_CURVE ( 'NONE', #11922, #89416, #62912, .T. ) ;
#55432=DIRECTION ( 'NONE',  ( -1.000000000000000000, 0.000000000000000000, 0.000000000000000000 ) ) ;
#55466=VECTOR ( 'NONE', #38861, 1000.000000000000000 ) ;
#55492=ORIENTED_EDGE ( 'NONE', *, *, #28792, .T. ) ;
#55496=ORIENTED_EDGE ( 'NONE', *, *, #254, .T. ) ;
#55564=VERTEX_POINT ( 'NONE', #15586 ) ;
#55588=LINE ( 'NONE', #63791, #2363 ) ;
#55699=VERTEX_POINT ( 'NONE', #53855 ) ;
#55742=AXIS2_PLACEMENT_3D ( 'NONE', #87263, #52250, #86372 ) ;
#55795=ADVANCED_FACE ( 'NONE', ( #49748 ), #15705, .T. ) ;
#55836=ORIENTED_EDGE ( 'NONE', *, *, #25941, .T. ) ;
#55846=CARTESIAN_POINT ( 'NONE',  ( 255.9983484187079910, 40.03750000000000142, 10.66800000000000104 ) ) ;
#55860=CIRCLE ( 'NONE', #38498, 4.762500000000002842 ) ;
#55880=AXIS2_PLACEMENT_3D ( 'NONE', #3667, #86790, #45862 ) ;
#55889=CARTESIAN_POINT ( 'NONE',  ( 241.3336515812914911, 40.03750000000000142, -2.032000000000000028 ) ) ;
#55904=EDGE_CURVE ( 'NONE', #18647, #30283, #62985, .T. ) ;
#55916=CARTESIAN_POINT ( 'NONE',  ( 210.5660000000000025, 52.73749999999999716, -37.80245750428454699 ) ) ;
#55923=ORIENTED_EDGE ( 'NONE', *, *, #83201, .T. ) ;
#55933=DIRECTION ( 'NONE',  ( 0.000000000000000000, 0.000000000000000000, 1.000000000000000000 ) ) ;
#55947=ORIENTED_EDGE ( 'NONE', *, *, #9589, .T. ) ;
#56068=CARTESIAN_POINT ( 'NONE',  ( 204.2160000000000082, 52.73749999999999716, -44.45000000000000284 ) ) ;
#56243=CARTESIAN_POINT ( 'NONE',  ( 210.5660000000000025, 52.73749999999999716, -49.21249999999999858 ) ) ;
#56310=AXIS2_PLACEMENT_3D ( 'NONE', #88609, #61320, #60419 ) ;
#56337=CARTESIAN_POINT ( 'NONE',  ( 241.3336515812914911, 40.03750000000000142, 10.66800000000000104 ) ) ;
#56399=CARTESIAN_POINT ( 'NONE',  ( 270.8910000000000196, 65.43750000000000000, 10.66800000000000104 ) ) ;
#56426=LINE ( 'NONE', #71875, #68673 ) ;
#56489=DIRECTION ( 'NONE',  ( 0.000000000000000000, 0.000000000000000000, -1.000000000000000000 ) ) ;
#56501=CARTESIAN_POINT ( 'NONE',  ( 199.3900000000000148, 52.73749999999999716, -53.97500000000000142 ) ) ;
#56529=VECTOR ( 'NONE', #6110, 1000.000000000000000 ) ;
#56565=DIRECTION ( 'NONE',  ( 0.000000000000000000, 0.000000000000000000, 1.000000000000000000 ) ) ;
#56579=ORIENTED_EDGE ( 'NONE', *, *, #76047, .T. ) ;
#56588=DIRECTION ( 'NONE',  ( -0.7071067811865444641, 0.000000000000000000, 0.7071067811865505703 ) ) ;
#56634=VERTEX_POINT ( 'NONE', #88663 ) ;
#56681=EDGE_LOOP ( 'NONE', ( #77174, #53567 ) ) ;
#56694=VECTOR ( 'NONE', #23726, 1000.000000000000000 ) ;
#56748=PLANE ( 'NONE',  #10068 ) ;
#56771=VERTEX_POINT ( 'NONE', #23984 ) ;
#56890=CARTESIAN_POINT ( 'NONE',  ( 183.5150000000000148, 14.63749999999999929, -52.38749999999999574 ) ) ;
#56918=CARTESIAN_POINT ( 'NONE',  ( 183.5150000000000148, 36.86249999999999716, -35.28456447661465489 ) ) ;
#56960=ADVANCED_FACE ( 'NONE', ( #40719 ), #54322, .F. ) ;
#56967=AXIS2_PLACEMENT_3D ( 'NONE', #23610, #36329, #65799 ) ;
#57090=ORIENTED_EDGE ( 'NONE', *, *, #41850, .F. ) ;
#57132=EDGE_LOOP ( 'NONE', ( #14571, #52473, #36019, #52278 ) ) ;
#57159=EDGE_CURVE ( 'NONE', #35999, #87914, #71141, .T. ) ;
#57192=ORIENTED_EDGE ( 'NONE', *, *, #41135, .T. ) ;
#57204=AXIS2_PLACEMENT_3D ( 'NONE', #43380, #27967, #35681 ) ;
#57231=ORIENTED_EDGE ( 'NONE', *, *, #23601, .F. ) ;
#57233=LINE ( 'NONE', #84978, #58660 ) ;
#57236=ORIENTED_EDGE ( 'NONE', *, *, #21202, .T. ) ;
#57247=CARTESIAN_POINT ( 'NONE',  ( 173.9899999999999807, 52.73749999999999716, -44.45000000000000284 ) ) ;
#57273=ADVANCED_FACE ( 'NONE', ( #24318 ), #16609, .T. ) ;
#57314=VERTEX_POINT ( 'NONE', #40156 ) ;
#57317=EDGE_LOOP ( 'NONE', ( #57090, #31914, #17091, #35183 ) ) ;
#57418=DIRECTION ( 'NONE',  ( 1.000000000000000000, 0.000000000000000000, 0.000000000000000000 ) ) ;
#57470=DIRECTION ( 'NONE',  ( 0.000000000000000000, 0.000000000000000000, -1.000000000000000000 ) ) ;
#57480=FACE_OUTER_BOUND ( 'NONE', #15, .T. ) ;
#57496=ORIENTED_EDGE ( 'NONE', *, *, #1386, .T. ) ;
#57593=VECTOR ( 'NONE', #66797, 1000.000000000000000 ) ;
#57629=LINE ( 'NONE', #66220, #59210 ) ;
#57669=SURFACE_SIDE_STYLE ('',( #64499 ) ) ;
#57712=DIRECTION ( 'NONE',  ( -1.000000000000000000, 0.000000000000000000, 0.000000000000000000 ) ) ;
#57764=LINE ( 'NONE', #72741, #52589 ) ;
#57784=EDGE_CURVE ( 'NONE', #35999, #88384, #82767, .T. ) ;
#57843=EDGE_CURVE ( 'NONE', #71161, #78791, #87682, .T. ) ;
#58009=DIRECTION ( 'NONE',  ( -1.000000000000000000, 0.000000000000000000, -2.108231265501709878E-16 ) ) ;
#58107=EDGE_LOOP ( 'NONE', ( #35265, #87327, #8113, #14335 ) ) ;
#58185=EDGE_CURVE ( 'NONE', #42451, #12839, #9577, .T. ) ;
#58194=ORIENTED_EDGE ( 'NONE', *, *, #85298, .T. ) ;
#58195=CARTESIAN_POINT ( 'NONE',  ( 177.1649999999999920, 25.81350000000000477, -7.937500000000000000 ) ) ;
#58217=EDGE_CURVE ( 'NONE', #73485, #8177, #66007, .T. ) ;
#58255=DIRECTION ( 'NONE',  ( 1.000000000000000000, 0.000000000000000000, 0.000000000000000000 ) ) ;
#58505=AXIS2_PLACEMENT_3D ( 'NONE', #27335, #20538, #62747 ) ;
#58638=CARTESIAN_POINT ( 'NONE',  ( 199.3900000000000148, 46.38749999999999574, -50.79999999999999716 ) ) ;
#58652=LINE ( 'NONE', #16450, #56694 ) ;
#58660=VECTOR ( 'NONE', #50423, 1000.000000000000000 ) ;
#58785=DIRECTION ( 'NONE',  ( 1.000000000000000000, 0.000000000000000000, 0.000000000000000000 ) ) ;
#58828=DIRECTION ( 'NONE',  ( 1.000000000000000000, 0.000000000000000000, 0.000000000000000000 ) ) ;
#58841=LINE ( 'NONE', #16200, #42260 ) ;
#58850=EDGE_CURVE ( 'NONE', #54417, #72244, #21545, .T. ) ;
#58855=CARTESIAN_POINT ( 'NONE',  ( 245.4909999999999854, 65.43750000000000000, -67.11950000000000216 ) ) ;
#58861=CARTESIAN_POINT ( 'NONE',  ( 270.8910000000000196, 65.43750000000000000, 10.66800000000000104 ) ) ;
#58882=CARTESIAN_POINT ( 'NONE',  ( 226.4410000000000025, 65.43750000000000000, -2.032000000000000028 ) ) ;
#58984=FACE_OUTER_BOUND ( 'NONE', #53707, .T. ) ;
#59041=ORIENTED_EDGE ( 'NONE', *, *, #23105, .T. ) ;
#59069=CARTESIAN_POINT ( 'NONE',  ( 248.6659999999999968, 52.73749999999999716, -2.903194600000015502 ) ) ;
#59084=DIRECTION ( 'NONE',  ( 0.000000000000000000, 0.000000000000000000, -1.000000000000000000 ) ) ;
#59104=DIRECTION ( 'NONE',  ( 2.098553464303459752E-16, 1.000000000000000000, 0.000000000000000000 ) ) ;
#59210=VECTOR ( 'NONE', #31710, 1000.000000000000000 ) ;
#59233=CIRCLE ( 'NONE', #73710, 3.968750000000520473 ) ;
#59261=LINE ( 'NONE', #45177, #72166 ) ;
#59298=CARTESIAN_POINT ( 'NONE',  ( 186.6899999999999977, 46.38749999999999574, -38.10000000000000142 ) ) ;
#59380=CARTESIAN_POINT ( 'NONE',  ( 210.5660000000000025, 52.73749999999999716, -44.45000000000000284 ) ) ;
#59520=ORIENTED_EDGE ( 'NONE', *, *, #21263, .T. ) ;
#59522=COLOUR_RGB ( '', 0.09019608, 0.27058824, 0.51372549) ;
#59526=CARTESIAN_POINT ( 'NONE',  ( 245.4909999999999854, 65.43750000000000000, -67.11950000000000216 ) ) ;
#59584=LINE ( 'NONE', #10560, #63887 ) ;
#59601=DIRECTION ( 'NONE',  ( 0.000000000000000000, 0.000000000000000000, 1.000000000000000000 ) ) ;
#59630=CARTESIAN_POINT ( 'NONE',  ( 183.5150000000000148, 14.63749999999999929, -47.62500000000000000 ) ) ;
#59638=ORIENTED_EDGE ( 'NONE', *, *, #37983, .T. ) ;
#59651=EDGE_CURVE ( 'NONE', #10845, #56771, #48990, .T. ) ;
#59672=CARTESIAN_POINT ( 'NONE',  ( 186.6899999999999977, 59.08750000000000568, -38.10000000000000142 ) ) ;
#59736=EDGE_CURVE ( 'NONE', #54672, #46304, #74914, .T. ) ;
#59797=DIRECTION ( 'NONE',  ( 0.000000000000000000, 0.000000000000000000, 1.000000000000000000 ) ) ;
#59807=EDGE_CURVE ( 'NONE', #71751, #62756, #9649, .T. ) ;
#59868=VERTEX_POINT ( 'NONE', #56337 ) ;
#59870=ORIENTED_EDGE ( 'NONE', *, *, #35304, .F. ) ;
#59895=VECTOR ( 'NONE', #3145, 1000.000000000000114 ) ;
#59900=VERTEX_POINT ( 'NONE', #69993 ) ;
#59902=EDGE_LOOP ( 'NONE', ( #32738, #26294, #43678, #31948 ) ) ;
#60035=VECTOR ( 'NONE', #15548, 1000.000000000000000 ) ;
#60039=DIRECTION ( 'NONE',  ( 1.000000000000000000, 0.000000000000000000, 0.000000000000000000 ) ) ;
#60085=VERTEX_POINT ( 'NONE', #38918 ) ;
#60135=CARTESIAN_POINT ( 'NONE',  ( 208.9149999999999920, 28.98850000000000193, -58.73749999999999716 ) ) ;
#60159=CARTESIAN_POINT ( 'NONE',  ( 270.8910000000000196, 40.03750000000000142, -67.11950000000000216 ) ) ;
#60365=CARTESIAN_POINT ( 'NONE',  ( 183.5150000000000148, 36.86249999999999716, -35.28456447661465489 ) ) ;
#60419=DIRECTION ( 'NONE',  ( 0.000000000000000000, 0.000000000000000000, 1.000000000000000000 ) ) ;
#60432=ADVANCED_FACE ( 'NONE', ( #23865, #87421 ), #18365, .T. ) ;
#60482=AXIS2_PLACEMENT_3D ( 'NONE', #54769, #6654, #21646 ) ;
#60492=EDGE_LOOP ( 'NONE', ( #7453, #65506, #81993, #79135 ) ) ;
#60497=DIRECTION ( 'NONE',  ( 0.000000000000000000, 0.000000000000000000, 1.000000000000000000 ) ) ;
#60498=PRODUCT ( 'Proximity Switch Housing', 'Proximity Switch Housing', '', ( #67193 ) ) ;
#60503=CARTESIAN_POINT ( 'NONE',  ( 183.5150000000000148, 68.61249999999999716, -53.61543552338530105 ) ) ;
#60512=LINE ( 'NONE', #19638, #68945 ) ;
#60615=DIRECTION ( 'NONE',  ( 0.000000000000000000, 0.000000000000000000, -1.000000000000000000 ) ) ;
#60687=DIRECTION ( 'NONE',  ( -1.000000000000000000, 0.000000000000000000, 0.000000000000000000 ) ) ;
#60700=ORIENTED_EDGE ( 'NONE', *, *, #65451, .F. ) ;
#60770=DIRECTION ( 'NONE',  ( 1.000000000000000000, 0.000000000000000000, 0.000000000000000000 ) ) ;
#60806=FACE_OUTER_BOUND ( 'NONE', #1102, .T. ) ;
#60825=ADVANCED_BREP_SHAPE_REPRESENTATION ( '', ( #80104, #50656 ), #7165 ) ;
#60850=EDGE_LOOP ( 'NONE', ( #14802, #26092 ) ) ;
#60961=PLANE ( 'NONE',  #26604 ) ;
#61009=EDGE_LOOP ( 'NONE', ( #71164, #7285, #32452, #39881, #50773 ) ) ;
#61064=EDGE_LOOP ( 'NONE', ( #73406, #49365, #10192, #10279 ) ) ;
#61105=AXIS2_PLACEMENT_3D ( 'NONE', #54000, #12709, #53095 ) ;
#61130=LINE ( 'NONE', #39779, #16111 ) ;
#61154=FACE_OUTER_BOUND ( 'NONE', #68986, .T. ) ;
#61170=ORIENTED_EDGE ( 'NONE', *, *, #75379, .F. ) ;
#61171=ORIENTED_EDGE ( 'NONE', *, *, #67623, .T. ) ;
#61173=AXIS2_PLACEMENT_3D ( 'NONE', #57247, #9570, #85449 ) ;
#61219=DIRECTION ( 'NONE',  ( 0.000000000000000000, 0.000000000000000000, -1.000000000000000000 ) ) ;
#61269=DIRECTION ( 'NONE',  ( 0.000000000000000000, 0.000000000000000000, 1.000000000000000000 ) ) ;
#61276=EDGE_LOOP ( 'NONE', ( #46538, #13830, #7617, #62354 ) ) ;
#61282=CARTESIAN_POINT ( 'NONE',  ( 263.3306968374159851, 52.73749999999999716, 10.66800000000000104 ) ) ;
#61300=DIRECTION ( 'NONE',  ( 0.000000000000000000, 0.000000000000000000, -1.000000000000000000 ) ) ;
#61320=DIRECTION ( 'NONE',  ( -1.000000000000000000, 0.000000000000000000, 0.000000000000000000 ) ) ;
#61431=VERTEX_POINT ( 'NONE', #37730 ) ;
#61507=CARTESIAN_POINT ( 'NONE',  ( 234.0013031625829854, 52.73749999999999716, -2.032000000000000028 ) ) ;
#61635=ORIENTED_EDGE ( 'NONE', *, *, #4776, .F. ) ;
#61823=ORIENTED_EDGE ( 'NONE', *, *, #81554, .F. ) ;
#61874=CARTESIAN_POINT ( 'NONE',  ( 226.4410000000000025, 65.43750000000000000, -63.94449999999999790 ) ) ;
#61900=DIRECTION ( 'NONE',  ( 0.7071067811865460184, 0.7071067811865489050, 0.000000000000000000 ) ) ;
#61972=DIRECTION ( 'NONE',  ( 0.000000000000000000, 1.000000000000000000, 0.000000000000000000 ) ) ;
#62091=DIRECTION ( 'NONE',  ( 0.7071067811865460184, 0.7071067811865489050, 0.000000000000000000 ) ) ;
#62109=ORIENTED_EDGE ( 'NONE', *, *, #66379, .F. ) ;
#62176=DIRECTION ( 'NONE',  ( 0.000000000000000000, 0.000000000000000000, -1.000000000000000000 ) ) ;
#62201=ORIENTED_EDGE ( 'NONE', *, *, #30094, .T. ) ;
#62226=DIRECTION ( 'NONE',  ( 0.000000000000000000, 0.000000000000000000, 1.000000000000000000 ) ) ;
#62299=CARTESIAN_POINT ( 'NONE',  ( 208.9149999999999920, 28.98850000000000193, -7.937500000000000000 ) ) ;
#62353=CARTESIAN_POINT ( 'NONE',  ( 210.2301280605339855, 25.81350000000000477, -7.937500000000000000 ) ) ;
#62354=ORIENTED_EDGE ( 'NONE', *, *, #41802, .F. ) ;
#62372=EDGE_CURVE ( 'NONE', #30425, #15176, #18678, .T. ) ;
#62430=EDGE_CURVE ( 'NONE', #84035, #9037, #69568, .T. ) ;
#62534=EDGE_LOOP ( 'NONE', ( #89035, #31636, #18772, #77630 ) ) ;
#62553=CIRCLE ( 'NONE', #11853, 8.928099999999993486 ) ;
#62625=ORIENTED_EDGE ( 'NONE', *, *, #16121, .F. ) ;
#62652=ORIENTED_EDGE ( 'NONE', *, *, #25587, .F. ) ;
#62667=CARTESIAN_POINT ( 'NONE',  ( 270.8910000000000196, 40.03750000000000142, 10.66800000000000104 ) ) ;
#62747=DIRECTION ( 'NONE',  ( 0.000000000000000000, 0.000000000000000000, 1.000000000000000000 ) ) ;
#62756=VERTEX_POINT ( 'NONE', #39057 ) ;
#62903=ORIENTED_EDGE ( 'NONE', *, *, #82703, .T. ) ;
#62912=CIRCLE ( 'NONE', #52699, 4.762500000000002842 ) ;
#62979=CARTESIAN_POINT ( 'NONE',  ( 199.3900000000000148, 59.08750000000000568, -50.79999999999999716 ) ) ;
#62985=CIRCLE ( 'NONE', #10781, 4.762500000000001066 ) ;
#63022=ADVANCED_FACE ( 'NONE', ( #77624, #14507 ), #7681, .F. ) ;
#63084=DIRECTION ( 'NONE',  ( 0.000000000000000000, 1.000000000000000000, 0.000000000000000000 ) ) ;
#63090=EDGE_LOOP ( 'NONE', ( #80053, #73104, #89249, #20056 ) ) ;
#63133=CARTESIAN_POINT ( 'NONE',  ( 208.9149999999999920, 28.98850000000000193, -7.937500000000000000 ) ) ;
#63221=PLANE ( 'NONE',  #86530 ) ;
#63344=PLANE ( 'NONE',  #30861 ) ;
#63535=CIRCLE ( 'NONE', #47630, 3.174999999999997158 ) ;
#63575=AXIS2_PLACEMENT_3D ( 'NONE', #47564, #68482, #80330 ) ;
#63689=CARTESIAN_POINT ( 'NONE',  ( 70.98999999999998067, 52.73749999999999716, -36.61250000000002558 ) ) ;
#63723=DIRECTION ( 'NONE',  ( 1.000000000000000000, -0.000000000000000000, 2.108231265501709878E-16 ) ) ;
#63791=CARTESIAN_POINT ( 'NONE',  ( 173.9900000000000091, 5.112500000000000711, -58.73749999999999716 ) ) ;
#63869=DIRECTION ( 'NONE',  ( 1.000000000000000000, 0.000000000000000000, 0.000000000000000000 ) ) ;
#63884=EDGE_LOOP ( 'NONE', ( #44911, #31620, #17519, #85779, #61635, #85008 ) ) ;
#63887=VECTOR ( 'NONE', #38705, 1000.000000000000000 ) ;
#63904=CARTESIAN_POINT ( 'NONE',  ( 210.2301280605339855, 25.81350000000000477, -7.937500000000000000 ) ) ;
#63944=ORIENTED_EDGE ( 'NONE', *, *, #75335, .T. ) ;
#64075=EDGE_CURVE ( 'NONE', #83557, #55564, #82505, .T. ) ;
#64168=EDGE_CURVE ( 'NONE', #8177, #9584, #1247, .T. ) ;
#64327=DIRECTION ( 'NONE',  ( 2.108231265501709878E-16, 5.463695987328529395E-16, -1.000000000000000000 ) ) ;
#64340=CARTESIAN_POINT ( 'NONE',  ( 70.98999999999998067, 52.73749999999999716, -44.45000000000002416 ) ) ;
#64343=VECTOR ( 'NONE', #28632, 1000.000000000000000 ) ;
#64382=LINE ( 'NONE', #36680, #38704 ) ;
#64424=VERTEX_POINT ( 'NONE', #77472 ) ;
#64462=VERTEX_POINT ( 'NONE', #17038 ) ;
#64499=SURFACE_STYLE_FILL_AREA ( #23624 ) ;
#64613=DIRECTION ( 'NONE',  ( -1.000000000000000000, 0.000000000000000000, 0.000000000000000000 ) ) ;
#64632=DIRECTION ( 'NONE',  ( 1.000000000000000000, 1.314511288311335947E-16, 0.000000000000000000 ) ) ;
#64643=EDGE_CURVE ( 'NONE', #83823, #30447, #17912, .T. ) ;
#64699=VERTEX_POINT ( 'NONE', #29220 ) ;
#64803=VERTEX_POINT ( 'NONE', #50986 ) ;
#64936=CARTESIAN_POINT ( 'NONE',  ( 248.6659999999999968, 52.73749999999999716, 10.66800000000000104 ) ) ;
#65076=CYLINDRICAL_SURFACE ( 'NONE', #11875, 7.837499999999996803 ) ;
#65151=ADVANCED_FACE ( 'NONE', ( #20059 ), #18256, .F. ) ;
#65166=VECTOR ( 'NONE', #42058, 1000.000000000000000 ) ;
#65230=CARTESIAN_POINT ( 'NONE',  ( 183.5150000000000148, 68.61249999999999716, -53.61543552338530105 ) ) ;
#65240=CARTESIAN_POINT ( 'NONE',  ( 183.5150000000000148, 36.86249999999999716, -53.61543552338530105 ) ) ;
#65243=VECTOR ( 'NONE', #79240, 1000.000000000000114 ) ;
#65284=FACE_OUTER_BOUND ( 'NONE', #65351, .T. ) ;
#65351=EDGE_LOOP ( 'NONE', ( #84843, #42645, #33911, #58194, #55492, #69447, #50220, #36082, #53679, #36124, #55923, #71188 ) ) ;
#65427=LINE ( 'NONE', #1868, #6662 ) ;
#65451=EDGE_CURVE ( 'NONE', #20936, #2985, #40269, .T. ) ;
#65506=ORIENTED_EDGE ( 'NONE', *, *, #54805, .T. ) ;
#65514=FILL_AREA_STYLE ('',( #86423 ) ) ;
#65600=ORIENTED_EDGE ( 'NONE', *, *, #44170, .F. ) ;
#65670=EDGE_CURVE ( 'NONE', #57314, #24899, #43399, .T. ) ;
#65680=ORIENTED_EDGE ( 'NONE', *, *, #8349, .T. ) ;
#65709=EDGE_CURVE ( 'NONE', #54710, #17992, #36156, .T. ) ;
#65795=VERTEX_POINT ( 'NONE', #3867 ) ;
#65798=ORIENTED_EDGE ( 'NONE', *, *, #53450, .F. ) ;
#65799=DIRECTION ( 'NONE',  ( 0.000000000000000000, 0.000000000000000000, 1.000000000000000000 ) ) ;
#65877=ORIENTED_EDGE ( 'NONE', *, *, #57843, .F. ) ;
#65935=ORIENTED_EDGE ( 'NONE', *, *, #13025, .F. ) ;
#65942=EDGE_CURVE ( 'NONE', #2982, #89416, #68331, .T. ) ;
#65944=VECTOR ( 'NONE', #73166, 1000.000000000000000 ) ;
#65967=CARTESIAN_POINT ( 'NONE',  ( 186.6899999999999977, 52.73749999999999716, -44.45000000000000284 ) ) ;
#66007=CIRCLE ( 'NONE', #68892, 3.174999999999997158 ) ;
#66028=VERTEX_POINT ( 'NONE', #88784 ) ;
#66047=ORIENTED_EDGE ( 'NONE', *, *, #64075, .F. ) ;
#66056=DIRECTION ( 'NONE',  ( 1.000000000000000000, 0.000000000000000000, 0.000000000000000000 ) ) ;
#66083=VECTOR ( 'NONE', #56588, 1000.000000000000114 ) ;
#66107=ADVANCED_FACE ( 'NONE', ( #12470 ), #74252, .T. ) ;
#66142=PRESENTATION_STYLE_ASSIGNMENT (( #85413 ) ) ;
#66220=CARTESIAN_POINT ( 'NONE',  ( 241.3336515812914911, 65.43750000000000000, -2.032000000000000028 ) ) ;
#66233=CARTESIAN_POINT ( 'NONE',  ( 186.6899999999999977, 59.08750000000000568, -50.79999999999999716 ) ) ;
#66239=ORIENTED_EDGE ( 'NONE', *, *, #43429, .F. ) ;
#66242=ORIENTED_EDGE ( 'NONE', *, *, #83533, .F. ) ;
#66379=EDGE_CURVE ( 'NONE', #59900, #69275, #59584, .T. ) ;
#66395=EDGE_CURVE ( 'NONE', #89416, #11922, #27618, .T. ) ;
#66428=EDGE_CURVE ( 'NONE', #18949, #32855, #86877, .T. ) ;
#66558=DIRECTION ( 'NONE',  ( 0.000000000000000000, -1.000000000000000000, 5.463695987328529395E-16 ) ) ;
#66576=DIRECTION ( 'NONE',  ( 0.000000000000000000, -1.000000000000000000, 0.000000000000000000 ) ) ;
#66602=EDGE_CURVE ( 'NONE', #14890, #62756, #36395, .T. ) ;
#66664=PLANE ( 'NONE',  #45846 ) ;
#66695=LINE ( 'NONE', #50838, #52617 ) ;
#66776=CYLINDRICAL_SURFACE ( 'NONE', #55880, 12.44599999999999795 ) ;
#66790=ORIENTED_EDGE ( 'NONE', *, *, #10937, .T. ) ;
#66797=DIRECTION ( 'NONE',  ( 0.000000000000000000, 1.000000000000000000, 0.000000000000000000 ) ) ;
#66877=DIRECTION ( 'NONE',  ( 1.000000000000000000, 0.000000000000000000, 0.000000000000000000 ) ) ;
#66882=DIRECTION ( 'NONE',  ( 0.000000000000000000, 0.000000000000000000, -1.000000000000000000 ) ) ;
#66932=LINE ( 'NONE', #73746, #17482 ) ;
#66938=ORIENTED_EDGE ( 'NONE', *, *, #12463, .T. ) ;
#66947=FACE_OUTER_BOUND ( 'NONE', #4580, .T. ) ;
#66967=FACE_OUTER_BOUND ( 'NONE', #80205, .T. ) ;
#66999=ORIENTED_EDGE ( 'NONE', *, *, #10919, .F. ) ;
#67005=EDGE_CURVE ( 'NONE', #19900, #84272, #12249, .T. ) ;
#67075=CARTESIAN_POINT ( 'NONE',  ( 210.2301280605339855, 25.81350000000000477, -58.73749999999999716 ) ) ;
#67107=AXIS2_PLACEMENT_3D ( 'NONE', #12435, #40123, #52824 ) ;
#67193=PRODUCT_CONTEXT ( 'NONE', #14364, 'mechanical' ) ;
#67202=DIRECTION ( 'NONE',  ( 1.000000000000000000, 0.000000000000000000, 0.000000000000000000 ) ) ;
#67272=ORIENTED_EDGE ( 'NONE', *, *, #66379, .T. ) ;
#67331=DIRECTION ( 'NONE',  ( 0.000000000000000000, 0.000000000000000000, 1.000000000000000000 ) ) ;
#67375=ADVANCED_FACE ( 'NONE', ( #51668, #17179 ), #50791, .F. ) ;
#67416=DIRECTION ( 'NONE',  ( 1.000000000000000000, 0.000000000000000000, 0.000000000000000000 ) ) ;
#67538=EDGE_CURVE ( 'NONE', #37523, #8565, #10536, .T. ) ;
#67565=CARTESIAN_POINT ( 'NONE',  ( 223.2659999999999911, 36.86249999999999716, -2.032000000000000028 ) ) ;
#67577=VECTOR ( 'NONE', #72719, 1000.000000000000000 ) ;
#67602=ORIENTED_EDGE ( 'NONE', *, *, #82969, .F. ) ;
#67623=EDGE_CURVE ( 'NONE', #37178, #19677, #47539, .T. ) ;
#67647=ORIENTED_EDGE ( 'NONE', *, *, #1493, .T. ) ;
#67684=CARTESIAN_POINT ( 'NONE',  ( 173.9900000000000091, 52.73749999999999716, -26.11912895322935313 ) ) ;
#67705=ORIENTED_EDGE ( 'NONE', *, *, #32887, .T. ) ;
#67732=CARTESIAN_POINT ( 'NONE',  ( 263.3306968374159851, 52.73749999999999716, -2.032000000000000028 ) ) ;
#67860=CARTESIAN_POINT ( 'NONE',  ( 234.0013031625829854, 52.73749999999999716, -2.032000000000000028 ) ) ;
#67891=PLANE ( 'NONE',  #70070 ) ;
#67954=AXIS2_PLACEMENT_3D ( 'NONE', #52072, #3067, #72109 ) ;
#68110=PLANE ( 'NONE',  #24110 ) ;
#68114=CARTESIAN_POINT ( 'NONE',  ( 183.5150000000000148, 68.61249999999999716, -35.28456447661459805 ) ) ;
#68138=CARTESIAN_POINT ( 'NONE',  ( 204.2160000000000082, 52.73749999999999716, -44.45000000000000284 ) ) ;
#68191=AXIS2_PLACEMENT_3D ( 'NONE', #39252, #11094, #58785 ) ;
#68227=AXIS2_PLACEMENT_3D ( 'NONE', #56890, #64613, #84631 ) ;
#68331=LINE ( 'NONE', #81974, #56529 ) ;
#68386=ORIENTED_EDGE ( 'NONE', *, *, #57159, .F. ) ;
#68457=CARTESIAN_POINT ( 'NONE',  ( 183.5150000000000148, 14.63749999999999929, -14.28749999999999964 ) ) ;
#68482=DIRECTION ( 'NONE',  ( -1.000000000000000000, 0.000000000000000000, 0.000000000000000000 ) ) ;
#68503=EDGE_LOOP ( 'NONE', ( #24004, #66239 ) ) ;
#68538=VECTOR ( 'NONE', #4243, 1000.000000000000000 ) ;
#68588=CARTESIAN_POINT ( 'NONE',  ( 183.5150000000000148, 36.86249999999999716, -35.28456447661465489 ) ) ;
#68590=DIRECTION ( 'NONE',  ( 0.000000000000000000, 0.000000000000000000, -1.000000000000000000 ) ) ;
#68609=PLANE ( 'NONE',  #81928 ) ;
#68620=DIRECTION ( 'NONE',  ( 0.000000000000000000, -1.000000000000000000, 0.000000000000000000 ) ) ;
#68673=VECTOR ( 'NONE', #9639, 1000.000000000000000 ) ;
#68697=DIRECTION ( 'NONE',  ( -1.000000000000000000, 0.000000000000000000, 0.000000000000000000 ) ) ;
#68722=LINE ( 'NONE', #12416, #42088 ) ;
#68762=EDGE_CURVE ( 'NONE', #82635, #71852, #1266, .T. ) ;
#68806=PLANE ( 'NONE',  #1642 ) ;
#68835=ORIENTED_EDGE ( 'NONE', *, *, #85933, .F. ) ;
#68842=ORIENTED_EDGE ( 'NONE', *, *, #71368, .F. ) ;
#68892=AXIS2_PLACEMENT_3D ( 'NONE', #47644, #33585, #39943 ) ;
#68896=EDGE_CURVE ( 'NONE', #30158, #28826, #17285, .T. ) ;
#68916=CARTESIAN_POINT ( 'NONE',  ( 210.2301280605339855, 25.81350000000000477, -58.73749999999999716 ) ) ;
#68945=VECTOR ( 'NONE', #47326, 1000.000000000000000 ) ;
#68986=EDGE_LOOP ( 'NONE', ( #71631, #36215 ) ) ;
#69012=VECTOR ( 'NONE', #26459, 1000.000000000000000 ) ;
#69051=ORIENTED_EDGE ( 'NONE', *, *, #41135, .F. ) ;
#69062=LINE ( 'NONE', #13209, #40309 ) ;
#69171=CARTESIAN_POINT ( 'NONE',  ( 234.0013031625829854, 52.73749999999999716, 10.66800000000000104 ) ) ;
#69253=FACE_OUTER_BOUND ( 'NONE', #86225, .T. ) ;
#69256=DIRECTION ( 'NONE',  ( 1.000000000000000000, 0.000000000000000000, 0.000000000000000000 ) ) ;
#69275=VERTEX_POINT ( 'NONE', #324 ) ;
#69350=AXIS2_PLACEMENT_3D ( 'NONE', #68457, #55244, #6671 ) ;
#69447=ORIENTED_EDGE ( 'NONE', *, *, #77880, .T. ) ;
#69460=VECTOR ( 'NONE', #81429, 1000.000000000000000 ) ;
#69522=DIRECTION ( 'NONE',  ( 0.000000000000000000, 0.000000000000000000, 1.000000000000000000 ) ) ;
#69568=LINE ( 'NONE', #89122, #69460 ) ;
#69572=AXIS2_PLACEMENT_3D ( 'NONE', #35497, #21897, #35052 ) ;
#69608=DIRECTION ( 'NONE',  ( 1.000000000000000000, 0.000000000000000000, 0.000000000000000000 ) ) ;
#69678=VERTEX_POINT ( 'NONE', #59298 ) ;
#69682=CARTESIAN_POINT ( 'NONE',  ( 223.2659999999999911, 52.73749999999999716, -44.45000000000000284 ) ) ;
#69739=ORIENTED_EDGE ( 'NONE', *, *, #7485, .T. ) ;
#69759=CIRCLE ( 'NONE', #17558, 4.762500000000001066 ) ;
#69855=VECTOR ( 'NONE', #32537, 1000.000000000000000 ) ;
#69875=LINE ( 'NONE', #15371, #9154 ) ;
#69963=CARTESIAN_POINT ( 'NONE',  ( 183.5150000000000148, 52.73749999999999716, -62.78087104677060637 ) ) ;
#69987=CARTESIAN_POINT ( 'NONE',  ( 263.3306968374159851, 52.73749999999999716, -2.032000000000000028 ) ) ;
#69993=CARTESIAN_POINT ( 'NONE',  ( 186.6899999999999977, 59.08750000000000568, -50.79999999999999716 ) ) ;
#70012=EDGE_CURVE ( 'NONE', #54782, #84272, #1909, .T. ) ;
#70025=FACE_OUTER_BOUND ( 'NONE', #41610, .T. ) ;
#70070=AXIS2_PLACEMENT_3D ( 'NONE', #45626, #60615, #73361 ) ;
#70159=FACE_OUTER_BOUND ( 'NONE', #1859, .T. ) ;
#70236=ORIENTED_EDGE ( 'NONE', *, *, #49557, .T. ) ;
#70244=CARTESIAN_POINT ( 'NONE',  ( 226.4410000000000025, 65.43750000000000000, -2.032000000000000028 ) ) ;
#70265=ORIENTED_EDGE ( 'NONE', *, *, #83201, .F. ) ;
#70355=ORIENTED_EDGE ( 'NONE', *, *, #11535, .F. ) ;
#70374=VECTOR ( 'NONE', #50444, 1000.000000000000000 ) ;
#70377=LINE ( 'NONE', #14971, #40349 ) ;
#70430=PLANE ( 'NONE',  #40322 ) ;
#70617=ORIENTED_EDGE ( 'NONE', *, *, #11437, .T. ) ;
#70675=DIRECTION ( 'NONE',  ( 1.825781832977094175E-16, -0.4999999999999998890, -0.8660254037844387076 ) ) ;
#70686=VECTOR ( 'NONE', #26309, 1000.000000000000000 ) ;
#70691=CARTESIAN_POINT ( 'NONE',  ( 213.1962561210690126, 52.73749999999999716, -44.45000000000000284 ) ) ;
#70704=VECTOR ( 'NONE', #50369, 1000.000000000000000 ) ;
#70725=CARTESIAN_POINT ( 'NONE',  ( 204.2160000000000082, 52.73749999999999716, -49.21249999999999858 ) ) ;
#70777=EDGE_LOOP ( 'NONE', ( #71596, #62625, #52789, #66790 ) ) ;
#70924=ORIENTED_EDGE ( 'NONE', *, *, #73227, .T. ) ;
#71043=CARTESIAN_POINT ( 'NONE',  ( 274.0659999999999741, 40.03750000000000142, -58.73749999999999716 ) ) ;
#71076=CARTESIAN_POINT ( 'NONE',  ( 223.2659999999999911, 52.73749999999999716, -44.45000000000000284 ) ) ;
#71137=CARTESIAN_POINT ( 'NONE',  ( 183.5150000000000148, 14.63749999999999929, -57.14999999999999858 ) ) ;
#71141=LINE ( 'NONE', #28904, #66083 ) ;
#71161=VERTEX_POINT ( 'NONE', #78245 ) ;
#71164=ORIENTED_EDGE ( 'NONE', *, *, #86587, .T. ) ;
#71188=ORIENTED_EDGE ( 'NONE', *, *, #46078, .T. ) ;
#71332=CARTESIAN_POINT ( 'NONE',  ( 263.3306968374159851, 52.73749999999999716, -2.032000000000000028 ) ) ;
#71368=EDGE_CURVE ( 'NONE', #6360, #19900, #49492, .T. ) ;
#71430=ORIENTED_EDGE ( 'NONE', *, *, #81443, .T. ) ;
#71433=EDGE_LOOP ( 'NONE', ( #65798, #21866, #74298, #17425 ) ) ;
#71596=ORIENTED_EDGE ( 'NONE', *, *, #50626, .T. ) ;
#71625=FACE_OUTER_BOUND ( 'NONE', #61276, .T. ) ;
#71631=ORIENTED_EDGE ( 'NONE', *, *, #84371, .T. ) ;
#71751=VERTEX_POINT ( 'NONE', #22124 ) ;
#71762=DIRECTION ( 'NONE',  ( 1.000000000000000000, 0.000000000000000000, 0.000000000000000000 ) ) ;
#71783=EDGE_CURVE ( 'NONE', #69275, #55699, #28009, .T. ) ;
#71831=AXIS2_PLACEMENT_3D ( 'NONE', #77468, #2067, #56565 ) ;
#71852=VERTEX_POINT ( 'NONE', #8864 ) ;
#71875=CARTESIAN_POINT ( 'NONE',  ( 226.4410000000000025, 65.43750000000000000, -63.94449999999999790 ) ) ;
#71897=( NAMED_UNIT ( * ) PLANE_ANGLE_UNIT ( ) SI_UNIT ( $, .RADIAN. ) );
#71924=LINE ( 'NONE', #44189, #52576 ) ;
#72043=ORIENTED_EDGE ( 'NONE', *, *, #28543, .F. ) ;
#72047=DIRECTION ( 'NONE',  ( 0.000000000000000000, 0.000000000000000000, 1.000000000000000000 ) ) ;
#72078=VECTOR ( 'NONE', #50862, 1000.000000000000000 ) ;
#72096=EDGE_LOOP ( 'NONE', ( #68842, #84337, #70617, #59041 ) ) ;
#72109=DIRECTION ( 'NONE',  ( 0.000000000000000000, 0.000000000000000000, 1.000000000000000000 ) ) ;
#72166=VECTOR ( 'NONE', #10666, 1000.000000000000000 ) ;
#72192=CYLINDRICAL_SURFACE ( 'NONE', #56967, 9.524999999999998579 ) ;
#72211=ORIENTED_EDGE ( 'NONE', *, *, #7131, .T. ) ;
#72238=EDGE_CURVE ( 'NONE', #21668, #71852, #68722, .T. ) ;
#72244=VERTEX_POINT ( 'NONE', #69171 ) ;
#72398=ORIENTED_EDGE ( 'NONE', *, *, #71783, .F. ) ;
#72400=AXIS2_PLACEMENT_3D ( 'NONE', #47777, #67331, #18747 ) ;
#72455=DIRECTION ( 'NONE',  ( 0.000000000000000000, 0.000000000000000000, 1.000000000000000000 ) ) ;
#72496=DIRECTION ( 'NONE',  ( 0.000000000000000000, 0.000000000000000000, 1.000000000000000000 ) ) ;
#72539=DIRECTION ( 'NONE',  ( -1.000000000000000000, 0.000000000000000000, 0.000000000000000000 ) ) ;
#72586=EDGE_LOOP ( 'NONE', ( #72043, #20177, #7223, #77961 ) ) ;
#72593=DIRECTION ( 'NONE',  ( 1.000000000000000000, -0.000000000000000000, 2.108231265501709878E-16 ) ) ;
#72675=CARTESIAN_POINT ( 'NONE',  ( 223.2659999999999911, 52.73749999999999716, -44.45000000000000284 ) ) ;
#72714=LINE ( 'NONE', #52226, #41426 ) ;
#72719=DIRECTION ( 'NONE',  ( -1.000000000000000000, 0.000000000000000000, 0.000000000000000000 ) ) ;
#72741=CARTESIAN_POINT ( 'NONE',  ( 274.0659999999999741, 40.03750000000000142, -7.937500000000000000 ) ) ;
#72743=ORIENTED_EDGE ( 'NONE', *, *, #75148, .T. ) ;
#72878=DIRECTION ( 'NONE',  ( -7.136255983449500255E-16, 0.000000000000000000, -1.000000000000000000 ) ) ;
#72910=CARTESIAN_POINT ( 'NONE',  ( 173.9900000000000091, 28.98850000000000193, -7.937500000000000000 ) ) ;
#72954=EDGE_CURVE ( 'NONE', #78791, #71161, #87105, .T. ) ;
#72978=AXIS2_PLACEMENT_3D ( 'NONE', #28807, #49674, #41073 ) ;
#73046=ADVANCED_FACE ( 'NONE', ( #58984 ), #84202, .F. ) ;
#73101=VECTOR ( 'NONE', #28012, 1000.000000000000000 ) ;
#73104=ORIENTED_EDGE ( 'NONE', *, *, #85933, .T. ) ;
#73131=CARTESIAN_POINT ( 'NONE',  ( 255.9983484187079910, 65.43750000000000000, 10.66800000000000104 ) ) ;
#73166=DIRECTION ( 'NONE',  ( 0.000000000000000000, 1.000000000000000000, 5.463695987328529395E-16 ) ) ;
#73227=EDGE_CURVE ( 'NONE', #61431, #65795, #53798, .T. ) ;
#73361=DIRECTION ( 'NONE',  ( 0.000000000000000000, -1.000000000000000000, 0.000000000000000000 ) ) ;
#73384=LINE ( 'NONE', #11154, #55466 ) ;
#73400=CARTESIAN_POINT ( 'NONE',  ( 183.5150000000000148, 14.63749999999999929, -9.525000000000000355 ) ) ;
#73406=ORIENTED_EDGE ( 'NONE', *, *, #13000, .T. ) ;
#73452=ORIENTED_EDGE ( 'NONE', *, *, #43429, .T. ) ;
#73477=LINE ( 'NONE', #38071, #22882 ) ;
#73479=FACE_OUTER_BOUND ( 'NONE', #22077, .T. ) ;
#73485=VERTEX_POINT ( 'NONE', #17568 ) ;
#73500=ORIENTED_EDGE ( 'NONE', *, *, #7131, .F. ) ;
#73546=DIRECTION ( 'NONE',  ( -0.8660254037844387076, -0.4999999999999998890, 0.000000000000000000 ) ) ;
#73569=EDGE_CURVE ( 'NONE', #54266, #66028, #61130, .T. ) ;
#73617=VECTOR ( 'NONE', #81891, 1000.000000000000000 ) ;
#73624=ORIENTED_EDGE ( 'NONE', *, *, #16518, .T. ) ;
#73626=CARTESIAN_POINT ( 'NONE',  ( 255.9983484187079910, 40.03750000000000142, -2.032000000000000028 ) ) ;
#73638=ORIENTED_EDGE ( 'NONE', *, *, #12175, .F. ) ;
#73668=CARTESIAN_POINT ( 'NONE',  ( 183.5150000000000148, 36.86249999999999716, -53.61543552338530105 ) ) ;
#73710=AXIS2_PLACEMENT_3D ( 'NONE', #23184, #78591, #16343 ) ;
#73746=CARTESIAN_POINT ( 'NONE',  ( 186.6899999999999977, 59.08750000000000568, -38.10000000000000142 ) ) ;
#73820=DIRECTION ( 'NONE',  ( 1.000000000000000000, 0.000000000000000000, 0.000000000000000000 ) ) ;
#73837=CIRCLE ( 'NONE', #34662, 8.928099999999993486 ) ;
#73903=PLANE ( 'NONE',  #81020 ) ;
#73946=CARTESIAN_POINT ( 'NONE',  ( 226.4410000000000025, 52.73749999999999716, -32.00399999999999778 ) ) ;
#74077=ADVANCED_FACE ( 'NONE', ( #21388 ), #12329, .T. ) ;
#74108=EDGE_CURVE ( 'NONE', #12759, #84665, #36807, .T. ) ;
#74168=DIRECTION ( 'NONE',  ( -1.314511288311335947E-16, 1.000000000000000000, 0.000000000000000000 ) ) ;
#74242=ADVANCED_FACE ( 'NONE', ( #53063 ), #18133, .T. ) ;
#74251=CARTESIAN_POINT ( 'NONE',  ( 226.4410000000000025, 52.73749999999999716, -44.45000000000000284 ) ) ;
#74252=PLANE ( 'NONE',  #82691 ) ;
#74269=CARTESIAN_POINT ( 'NONE',  ( 177.1649999999999920, 25.81350000000000477, -7.937500000000000000 ) ) ;
#74298=ORIENTED_EDGE ( 'NONE', *, *, #55400, .T. ) ;
#74316=ORIENTED_EDGE ( 'NONE', *, *, #80354, .T. ) ;
#74351=VERTEX_POINT ( 'NONE', #74450 ) ;
#74355=DIRECTION ( 'NONE',  ( 0.000000000000000000, -1.000000000000000000, 5.463695987328529395E-16 ) ) ;
#74424=ORIENTED_EDGE ( 'NONE', *, *, #18201, .F. ) ;
#74450=CARTESIAN_POINT ( 'NONE',  ( 241.3336515812914911, 65.43750000000000000, -2.032000000000000028 ) ) ;
#74462=EDGE_CURVE ( 'NONE', #47225, #64699, #53970, .T. ) ;
#74468=ADVANCED_FACE ( 'NONE', ( #60806 ), #54416, .T. ) ;
#74474=CARTESIAN_POINT ( 'NONE',  ( 257.5940999999999690, 52.73749999999999716, -2.903194600000015502 ) ) ;
#74481=AXIS2_PLACEMENT_3D ( 'NONE', #83322, #76952, #56489 ) ;
#74555=DIRECTION ( 'NONE',  ( 0.000000000000000000, 0.000000000000000000, 1.000000000000000000 ) ) ;
#74626=AXIS2_PLACEMENT_3D ( 'NONE', #72675, #52186, #10440 ) ;
#74683=LINE ( 'NONE', #12464, #35008 ) ;
#74733=FACE_OUTER_BOUND ( 'NONE', #8064, .T. ) ;
#74735=CARTESIAN_POINT ( 'NONE',  ( 204.2160000000000082, 52.73749999999999716, -47.62500000000000000 ) ) ;
#74812=ORIENTED_EDGE ( 'NONE', *, *, #46078, .F. ) ;
#74848=AXIS2_PLACEMENT_3D ( 'NONE', #82345, #74168, #11948 ) ;
#74864=DIRECTION ( 'NONE',  ( 0.000000000000000000, 0.000000000000000000, -1.000000000000000000 ) ) ;
#74898=DIRECTION ( 'NONE',  ( 0.000000000000000000, 0.000000000000000000, -1.000000000000000000 ) ) ;
#74914=CIRCLE ( 'NONE', #28475, 9.524999999999998579 ) ;
#74996=DIRECTION ( 'NONE',  ( 0.000000000000000000, 0.000000000000000000, 1.000000000000000000 ) ) ;
#75062=CARTESIAN_POINT ( 'NONE',  ( 226.4410000000000025, 52.73749999999999716, -44.45000000000000284 ) ) ;
#75063=PLANE ( 'NONE',  #74848 ) ;
#75074=AXIS2_PLACEMENT_3D ( 'NONE', #74251, #17931, #12025 ) ;
#75105=CARTESIAN_POINT ( 'NONE',  ( 183.5150000000000148, 52.73749999999999716, -62.78087104677060637 ) ) ;
#75148=EDGE_CURVE ( 'NONE', #57314, #38623, #13905, .T. ) ;
#75182=CARTESIAN_POINT ( 'NONE',  ( 226.4410000000000025, 40.03750000000000142, 10.66800000000000104 ) ) ;
#75190=ORIENTED_EDGE ( 'NONE', *, *, #81443, .F. ) ;
#75335=EDGE_CURVE ( 'NONE', #78380, #31104, #86537, .T. ) ;
#75363=DIRECTION ( 'NONE',  ( 0.000000000000000000, -1.000000000000000000, 0.000000000000000000 ) ) ;
#75379=EDGE_CURVE ( 'NONE', #54417, #6675, #40140, .T. ) ;
#75388=DIRECTION ( 'NONE',  ( 0.000000000000000000, 0.000000000000000000, -1.000000000000000000 ) ) ;
#75416=CARTESIAN_POINT ( 'NONE',  ( 274.0659999999999741, 40.03750000000000142, -58.73749999999999716 ) ) ;
#75425=EDGE_LOOP ( 'NONE', ( #50342, #45130, #35520, #57192 ) ) ;
#75450=CARTESIAN_POINT ( 'NONE',  ( 173.9900000000000091, 52.73749999999999716, -62.78087104677060637 ) ) ;
#75481=DIRECTION ( 'NONE',  ( -0.7071067811865490160, 0.7071067811865461294, 0.000000000000000000 ) ) ;
#75527=CARTESIAN_POINT ( 'NONE',  ( 248.6659999999999968, 52.73749999999999716, 10.66800000000000104 ) ) ;
#75540=CIRCLE ( 'NONE', #36389, 6.647542495715439870 ) ;
#75660=CARTESIAN_POINT ( 'NONE',  ( 213.4642805167760002, 52.73749999999999716, -44.45000000000000284 ) ) ;
#75808=CARTESIAN_POINT ( 'NONE',  ( 205.0097499999990305, 52.73749999999999716, -44.45000000000000284 ) ) ;
#75841=ADVANCED_FACE ( 'NONE', ( #37370 ), #65076, .T. ) ;
#75937=ORIENTED_EDGE ( 'NONE', *, *, #1029, .T. ) ;
#76007=ORIENTED_EDGE ( 'NONE', *, *, #55333, .T. ) ;
#76029=LINE ( 'NONE', #33801, #35975 ) ;
#76047=EDGE_CURVE ( 'NONE', #12839, #15555, #66695, .T. ) ;
#76098=EDGE_CURVE ( 'NONE', #64699, #28622, #17664, .T. ) ;
#76127=DIRECTION ( 'NONE',  ( -2.108231265501709878E-16, 0.000000000000000000, 1.000000000000000000 ) ) ;
#76189=EDGE_LOOP ( 'NONE', ( #109, #84506, #30924, #67272 ) ) ;
#76205=ADVANCED_FACE ( 'NONE', ( #81251 ), #80226, .T. ) ;
#76267=AXIS2_PLACEMENT_3D ( 'NONE', #33605, #27230, #61300 ) ;
#76295=ORIENTED_EDGE ( 'NONE', *, *, #76740, .F. ) ;
#76348=ORIENTED_EDGE ( 'NONE', *, *, #40259, .F. ) ;
#76445=PLANE ( 'NONE',  #36653 ) ;
#76492=DIRECTION ( 'NONE',  ( -1.000000000000000000, 0.000000000000000000, 0.000000000000000000 ) ) ;
#76524=CARTESIAN_POINT ( 'NONE',  ( 183.5150000000000148, 52.73749999999999716, -26.11912895322935313 ) ) ;
#76543=VECTOR ( 'NONE', #77755, 1000.000000000000000 ) ;
#76569=CARTESIAN_POINT ( 'NONE',  ( 241.3336515812914911, 65.43750000000000000, 10.66800000000000104 ) ) ;
#76592=DIRECTION ( 'NONE',  ( 0.000000000000000000, -0.8660254037844387076, 0.4999999999999998890 ) ) ;
#76693=EDGE_CURVE ( 'NONE', #3831, #71161, #10739, .T. ) ;
#76708=ORIENTED_EDGE ( 'NONE', *, *, #86010, .T. ) ;
#76740=EDGE_CURVE ( 'NONE', #74351, #12839, #43468, .T. ) ;
#76833=CARTESIAN_POINT ( 'NONE',  ( 213.1962561210690126, 52.73749999999999716, -47.62500000000000000 ) ) ;
#76948=CARTESIAN_POINT ( 'NONE',  ( 223.2659999999999911, 52.73749999999999716, -56.89600000000000080 ) ) ;
#76952=DIRECTION ( 'NONE',  ( 1.000000000000000000, 0.000000000000000000, 0.000000000000000000 ) ) ;
#76956=VERTEX_POINT ( 'NONE', #45685 ) ;
#76990=AXIS2_PLACEMENT_3D ( 'NONE', #64936, #9978, #30420 ) ;
#76998=ORIENTED_EDGE ( 'NONE', *, *, #3471, .T. ) ;
#77012=DIRECTION ( 'NONE',  ( 0.000000000000000000, 0.000000000000000000, -1.000000000000000000 ) ) ;
#77090=EDGE_CURVE ( 'NONE', #78558, #47032, #45144, .T. ) ;
#77131=APPLICATION_CONTEXT ( 'automotive_design' ) ;
#77135=CARTESIAN_POINT ( 'NONE',  ( 234.0013031625829854, 52.73749999999999716, 10.66800000000000104 ) ) ;
#77146=FACE_OUTER_BOUND ( 'NONE', #22950, .T. ) ;
#77174=ORIENTED_EDGE ( 'NONE', *, *, #66395, .F. ) ;
#77184=ADVANCED_FACE ( 'NONE', ( #66947, #53284 ), #4729, .T. ) ;
#77222=CARTESIAN_POINT ( 'NONE',  ( 173.9900000000000091, 36.86249999999999716, -35.28456447661465489 ) ) ;
#77228=PLANE ( 'NONE',  #50129 ) ;
#77240=VECTOR ( 'NONE', #83274, 1000.000000000000000 ) ;
#77289=EDGE_CURVE ( 'NONE', #56771, #76956, #48265, .T. ) ;
#77290=CARTESIAN_POINT ( 'NONE',  ( 226.4410000000000025, 40.03750000000000142, 10.66800000000000104 ) ) ;
#77338=FACE_OUTER_BOUND ( 'NONE', #55338, .T. ) ;
#77355=ADVANCED_FACE ( 'NONE', ( #14228 ), #76445, .F. ) ;
#77416=EDGE_LOOP ( 'NONE', ( #574, #51080, #40106, #81423 ) ) ;
#77468=CARTESIAN_POINT ( 'NONE',  ( 223.2659999999999911, 52.73749999999999716, -44.45000000000000284 ) ) ;
#77472=CARTESIAN_POINT ( 'NONE',  ( 259.3340000000000032, 52.73749999999999716, 10.66800000000000104 ) ) ;
#77492=CARTESIAN_POINT ( 'NONE',  ( 186.6899999999999977, 46.38749999999999574, -50.79999999999999716 ) ) ;
#77624=FACE_OUTER_BOUND ( 'NONE', #6379, .T. ) ;
#77630=ORIENTED_EDGE ( 'NONE', *, *, #42075, .T. ) ;
#77698=ORIENTED_EDGE ( 'NONE', *, *, #74108, .F. ) ;
#77699=CARTESIAN_POINT ( 'NONE',  ( 173.9900000000000091, 28.98850000000000193, -7.937500000000000000 ) ) ;
#77753=FACE_OUTER_BOUND ( 'NONE', #63884, .T. ) ;
#77755=DIRECTION ( 'NONE',  ( 0.000000000000000000, 0.000000000000000000, -1.000000000000000000 ) ) ;
#77756=FACE_BOUND ( 'NONE', #28851, .T. ) ;
#77880=EDGE_CURVE ( 'NONE', #25134, #60085, #69875, .T. ) ;
#77949=FACE_OUTER_BOUND ( 'NONE', #53942, .T. ) ;
#77955=EDGE_LOOP ( 'NONE', ( #87558, #81926, #9637, #88584 ) ) ;
#77961=ORIENTED_EDGE ( 'NONE', *, *, #67538, .F. ) ;
#77991=VECTOR ( 'NONE', #14351, 1000.000000000000000 ) ;
#78038=DIRECTION ( 'NONE',  ( 0.4999999999999998890, -0.8660254037844387076, 0.000000000000000000 ) ) ;
#78101=EDGE_CURVE ( 'NONE', #31104, #71751, #81181, .T. ) ;
#78140=DIRECTION ( 'NONE',  ( 0.000000000000000000, 0.000000000000000000, -1.000000000000000000 ) ) ;
#78177=VERTEX_POINT ( 'NONE', #67075 ) ;
#78245=CARTESIAN_POINT ( 'NONE',  ( 199.3900000000000148, 52.73749999999999716, -41.27499999999999858 ) ) ;
#78247=( GEOMETRIC_REPRESENTATION_CONTEXT ( 3 ) GLOBAL_UNCERTAINTY_ASSIGNED_CONTEXT ( ( #36914 ) ) GLOBAL_UNIT_ASSIGNED_CONTEXT ( ( #36918, #10990, #37365 ) ) REPRESENTATION_CONTEXT ( 'NONE', 'WORKASPACE' ) );
#78268=FACE_OUTER_BOUND ( 'NONE', #8158, .T. ) ;
#78320=CIRCLE ( 'NONE', #11587, 4.762500000000002842 ) ;
#78327=FACE_OUTER_BOUND ( 'NONE', #12522, .T. ) ;
#78373=PRODUCT_DEFINITION_FORMATION_WITH_SPECIFIED_SOURCE ( 'ANY', '', #60498, .NOT_KNOWN. ) ;
#78380=VERTEX_POINT ( 'NONE', #35232 ) ;
#78424=VECTOR ( 'NONE', #34583, 1000.000000000000000 ) ;
#78432=ORIENTED_EDGE ( 'NONE', *, *, #4790, .F. ) ;
#78556=AXIS2_PLACEMENT_3D ( 'NONE', #45817, #73546, #32204 ) ;
#78558=VERTEX_POINT ( 'NONE', #45164 ) ;
#78591=DIRECTION ( 'NONE',  ( -1.000000000000000000, 0.000000000000000000, 0.000000000000000000 ) ) ;
#78593=CARTESIAN_POINT ( 'NONE',  ( 199.3900000000000148, 52.73749999999999716, -44.45000000000000284 ) ) ;
#78676=DIRECTION ( 'NONE',  ( 0.000000000000000000, 0.000000000000000000, 1.000000000000000000 ) ) ;
#78729=DIRECTION ( 'NONE',  ( 0.000000000000000000, 0.000000000000000000, -1.000000000000000000 ) ) ;
#78751=VECTOR ( 'NONE', #13353, 1000.000000000000000 ) ;
#78791=VERTEX_POINT ( 'NONE', #89214 ) ;
#78838=DIRECTION ( 'NONE',  ( -1.000000000000000000, 0.000000000000000000, 0.000000000000000000 ) ) ;
#78954=VECTOR ( 'NONE', #46894, 1000.000000000000000 ) ;
#79077=ORIENTED_EDGE ( 'NONE', *, *, #84371, .F. ) ;
#79135=ORIENTED_EDGE ( 'NONE', *, *, #76693, .F. ) ;
#79230=AXIS2_PLACEMENT_3D ( 'NONE', #70691, #36166, #83885 ) ;
#79240=DIRECTION ( 'NONE',  ( 0.7071067811865344721, 8.659560562355082002E-17, 0.7071067811865604513 ) ) ;
#79377=CARTESIAN_POINT ( 'NONE',  ( 270.8910000000000196, 65.43750000000000000, -2.032000000000000028 ) ) ;
#79444=LINE ( 'NONE', #51696, #9678 ) ;
#79476=DIRECTION ( 'NONE',  ( -0.000000000000000000, -0.000000000000000000, -1.000000000000000000 ) ) ;
#79517=ORIENTED_EDGE ( 'NONE', *, *, #58185, .F. ) ;
#79588=CONICAL_SURFACE ( 'NONE', #43310, 10.66800000000000992, 0.02993239667170383839 ) ;
#79725=DIRECTION ( 'NONE',  ( -1.000000000000000000, 0.000000000000000000, 0.000000000000000000 ) ) ;
#79730=DIRECTION ( 'NONE',  ( -1.000000000000000000, 0.000000000000000000, 0.000000000000000000 ) ) ;
#79798=LINE ( 'NONE', #81589, #51582 ) ;
#79806=CIRCLE ( 'NONE', #68191, 8.928099999999993486 ) ;
#79966=ADVANCED_FACE ( 'NONE', ( #41786 ), #54953, .T. ) ;
#79977=CARTESIAN_POINT ( 'NONE',  ( 210.5660000000000025, 52.73749999999999716, -51.09754249571540186 ) ) ;
#80001=DIRECTION ( 'NONE',  ( -1.000000000000000000, 0.000000000000000000, 0.000000000000000000 ) ) ;
#80006=ORIENTED_EDGE ( 'NONE', *, *, #4941, .F. ) ;
#80053=ORIENTED_EDGE ( 'NONE', *, *, #85437, .F. ) ;
#80104=MANIFOLD_SOLID_BREP ( 'Stock-BR-Y-104-1', #15549 ) ;
#80205=EDGE_LOOP ( 'NONE', ( #81581, #79077, #72211, #41650 ) ) ;
#80226=CONICAL_SURFACE ( 'NONE', #35275, 3.968750000000520473, 0.7853981633974667087 ) ;
#80259=ADVANCED_FACE ( 'NONE', ( #49281 ), #30973, .T. ) ;
#80281=ORIENTED_EDGE ( 'NONE', *, *, #54541, .F. ) ;
#80330=DIRECTION ( 'NONE',  ( 0.000000000000000000, 0.000000000000000000, 1.000000000000000000 ) ) ;
#80345=DIRECTION ( 'NONE',  ( 0.000000000000000000, -1.000000000000000000, 0.000000000000000000 ) ) ;
#80354=EDGE_CURVE ( 'NONE', #8565, #37523, #55860, .T. ) ;
#80424=FACE_OUTER_BOUND ( 'NONE', #75425, .T. ) ;
#80429=LINE ( 'NONE', #67684, #15406 ) ;
#80527=CARTESIAN_POINT ( 'NONE',  ( 234.0013031625829854, 52.73749999999999716, -2.032000000000000028 ) ) ;
#80530=FACE_OUTER_BOUND ( 'NONE', #38978, .T. ) ;
#80638=ORIENTED_EDGE ( 'NONE', *, *, #31867, .T. ) ;
#80652=FACE_OUTER_BOUND ( 'NONE', #72586, .T. ) ;
#80656=DIRECTION ( 'NONE',  ( -1.000000000000000000, 0.000000000000000000, -2.108231265501709878E-16 ) ) ;
#80674=ORIENTED_EDGE ( 'NONE', *, *, #71783, .T. ) ;
#80684=ORIENTED_EDGE ( 'NONE', *, *, #6410, .T. ) ;
#80688=AXIS2_PLACEMENT_3D ( 'NONE', #68138, #39077, #68590 ) ;
#80689=ORIENTED_EDGE ( 'NONE', *, *, #48222, .T. ) ;
#80713=VECTOR ( 'NONE', #38383, 1000.000000000000000 ) ;
#80723=FACE_OUTER_BOUND ( 'NONE', #68503, .T. ) ;
#80751=ORIENTED_EDGE ( 'NONE', *, *, #85437, .T. ) ;
#80761=DIRECTION ( 'NONE',  ( 0.000000000000000000, 0.000000000000000000, 1.000000000000000000 ) ) ;
#80857=CYLINDRICAL_SURFACE ( 'NONE', #53916, 8.928099999999993486 ) ;
#80961=LINE ( 'NONE', #33684, #49599 ) ;
#81020=AXIS2_PLACEMENT_3D ( 'NONE', #39808, #11687, #74355 ) ;
#81040=EDGE_LOOP ( 'NONE', ( #68835, #47814, #28267, #11981 ) ) ;
#81072=CARTESIAN_POINT ( 'NONE',  ( 223.2659999999999911, 52.73749999999999716, -44.45000000000000284 ) ) ;
#81085=CARTESIAN_POINT ( 'NONE',  ( 173.9900000000000091, 28.98850000000000193, -58.73749999999999716 ) ) ;
#81181=LINE ( 'NONE', #19826, #4869 ) ;
#81251=FACE_OUTER_BOUND ( 'NONE', #77416, .T. ) ;
#81263=CARTESIAN_POINT ( 'NONE',  ( 248.6659999999999968, 52.73749999999999716, -10.97647784993501396 ) ) ;
#81300=LINE ( 'NONE', #81742, #33520 ) ;
#81336=VECTOR ( 'NONE', #24639, 1000.000000000000114 ) ;
#81351=CARTESIAN_POINT ( 'NONE',  ( 177.1649999999999920, 5.112500000000000711, -58.73749999999999716 ) ) ;
#81389=ADVANCED_FACE ( 'NONE', ( #28876 ), #48582, .T. ) ;
#81423=ORIENTED_EDGE ( 'NONE', *, *, #68762, .F. ) ;
#81429=DIRECTION ( 'NONE',  ( 0.000000000000000000, -1.000000000000000000, 0.000000000000000000 ) ) ;
#81443=EDGE_CURVE ( 'NONE', #31184, #3831, #6526, .T. ) ;
#81468=CARTESIAN_POINT ( 'NONE',  ( 270.8910000000000196, 40.03750000000000142, -67.11950000000000216 ) ) ;
#81474=VECTOR ( 'NONE', #2742, 1000.000000000000000 ) ;
#81554=EDGE_CURVE ( 'NONE', #87657, #84035, #45154, .T. ) ;
#81572=PLANE ( 'NONE',  #2428 ) ;
#81581=ORIENTED_EDGE ( 'NONE', *, *, #30094, .F. ) ;
#81589=CARTESIAN_POINT ( 'NONE',  ( 219.9639999999999986, 40.03750000000000142, -58.73749999999999716 ) ) ;
#81597=ORIENTED_EDGE ( 'NONE', *, *, #59651, .T. ) ;
#81640=CARTESIAN_POINT ( 'NONE',  ( 183.5150000000000148, 52.73749999999999716, -62.78087104677060637 ) ) ;
#81742=CARTESIAN_POINT ( 'NONE',  ( 173.9900000000000091, 5.112500000000000711, -7.937500000000000000 ) ) ;
#81824=CARTESIAN_POINT ( 'NONE',  ( 210.5660000000000025, 52.73749999999999716, -44.45000000000000284 ) ) ;
#81883=ORIENTED_EDGE ( 'NONE', *, *, #57843, .T. ) ;
#81891=DIRECTION ( 'NONE',  ( 0.000000000000000000, 0.000000000000000000, 1.000000000000000000 ) ) ;
#81926=ORIENTED_EDGE ( 'NONE', *, *, #85503, .T. ) ;
#81928=AXIS2_PLACEMENT_3D ( 'NONE', #5942, #62226, #89046 ) ;
#81951=ORIENTED_EDGE ( 'NONE', *, *, #45978, .F. ) ;
#81974=CARTESIAN_POINT ( 'NONE',  ( 183.5150000000000148, 14.63749999999999929, -47.62500000000000000 ) ) ;
#81992=ORIENTED_EDGE ( 'NONE', *, *, #31313, .T. ) ;
#81993=ORIENTED_EDGE ( 'NONE', *, *, #72954, .T. ) ;
#81994=VERTEX_POINT ( 'NONE', #60135 ) ;
#82092=DIRECTION ( 'NONE',  ( 0.000000000000000000, 0.000000000000000000, 1.000000000000000000 ) ) ;
#82129=VECTOR ( 'NONE', #55358, 1000.000000000000000 ) ;
#82154=CARTESIAN_POINT ( 'NONE',  ( 183.5150000000000148, 68.61249999999999716, -35.28456447661459805 ) ) ;
#82206=CYLINDRICAL_SURFACE ( 'NONE', #79230, 3.174999999999997158 ) ;
#82343=CARTESIAN_POINT ( 'NONE',  ( 221.2791280605339921, 36.86249999999999716, -7.937500000000000000 ) ) ;
#82345=CARTESIAN_POINT ( 'NONE',  ( 274.0659999999999741, 36.86249999999999716, -7.937500000000000000 ) ) ;
#82356=FACE_OUTER_BOUND ( 'NONE', #39836, .T. ) ;
#82371=DIRECTION ( 'NONE',  ( 0.000000000000000000, 0.000000000000000000, 1.000000000000000000 ) ) ;
#82392=CIRCLE ( 'NONE', #37382, 12.44599999999999795 ) ;
#82454=LINE ( 'NONE', #56501, #49449 ) ;
#82486=CARTESIAN_POINT ( 'NONE',  ( 173.9900000000000091, 68.61249999999999716, -53.61543552338530105 ) ) ;
#82501=DIRECTION ( 'NONE',  ( -0.02992792722492364568, 3.665114028111763974E-18, 0.9995520592605569021 ) ) ;
#82505=CIRCLE ( 'NONE', #67954, 7.837499999999996803 ) ;
#82526=DIRECTION ( 'NONE',  ( 1.000000000000000000, 0.000000000000000000, 2.108231265501709878E-16 ) ) ;
#82574=VECTOR ( 'NONE', #45591, 1000.000000000000000 ) ;
#82623=ADVANCED_FACE ( 'NONE', ( #20070 ), #14146, .F. ) ;
#82635=VERTEX_POINT ( 'NONE', #86325 ) ;
#82689=ORIENTED_EDGE ( 'NONE', *, *, #43091, .F. ) ;
#82691=AXIS2_PLACEMENT_3D ( 'NONE', #12026, #67416, #40155 ) ;
#82703=EDGE_CURVE ( 'NONE', #4611, #56634, #65427, .T. ) ;
#82719=ORIENTED_EDGE ( 'NONE', *, *, #77289, .F. ) ;
#82762=AXIS2_PLACEMENT_3D ( 'NONE', #4201, #25083, #52747 ) ;
#82767=LINE ( 'NONE', #88678, #662 ) ;
#82777=LINE ( 'NONE', #76833, #30956 ) ;
#82794=LINE ( 'NONE', #46875, #73617 ) ;
#82881=DIRECTION ( 'NONE',  ( 0.000000000000000000, 0.000000000000000000, 1.000000000000000000 ) ) ;
#82969=EDGE_CURVE ( 'NONE', #47477, #44015, #25876, .T. ) ;
#83047=AXIS2_PLACEMENT_3D ( 'NONE', #44864, #72593, #10356 ) ;
#83080=ADVANCED_FACE ( 'NONE', ( #84340 ), #68110, .T. ) ;
#83086=ADVANCED_FACE ( 'NONE', ( #35255 ), #82206, .T. ) ;
#83201=EDGE_CURVE ( 'NONE', #24899, #12759, #23004, .T. ) ;
#83203=CARTESIAN_POINT ( 'NONE',  ( 219.9639999999999986, 40.03750000000000142, -7.937500000000000000 ) ) ;
#83274=DIRECTION ( 'NONE',  ( 1.000000000000000000, 1.314511288311335947E-16, 0.000000000000000000 ) ) ;
#83322=CARTESIAN_POINT ( 'NONE',  ( 183.5150000000000148, 52.73749999999999716, -44.45000000000000284 ) ) ;
#83347=DIRECTION ( 'NONE',  ( -1.000000000000000000, 0.000000000000000000, -2.108231265501709878E-16 ) ) ;
#83392=AXIS2_PLACEMENT_3D ( 'NONE', #40707, #82526, #76127 ) ;
#83438=LINE ( 'NONE', #21214, #73101 ) ;
#83533=EDGE_CURVE ( 'NONE', #84299, #47032, #18182, .T. ) ;
#83557=VERTEX_POINT ( 'NONE', #28798 ) ;
#83559=AXIS2_PLACEMENT_3D ( 'NONE', #32139, #4896, #32585 ) ;
#83602=DIRECTION ( 'NONE',  ( 0.000000000000000000, 0.000000000000000000, -1.000000000000000000 ) ) ;
#83662=DIRECTION ( 'NONE',  ( -1.000000000000000000, 0.000000000000000000, 5.463695987328529395E-16 ) ) ;
#83718=CARTESIAN_POINT ( 'NONE',  ( 173.9900000000000091, 28.98850000000000193, -7.937500000000000000 ) ) ;
#83719=VECTOR ( 'NONE', #84769, 1000.000000000000000 ) ;
#83789=CARTESIAN_POINT ( 'NONE',  ( 213.1962561210690126, 52.73749999999999716, -44.45000000000000284 ) ) ;
#83798=CIRCLE ( 'NONE', #40266, 3.968750000000520473 ) ;
#83800=DIRECTION ( 'NONE',  ( 1.825781832977096147E-16, 0.5000000000000003331, -0.8660254037844384856 ) ) ;
#83823=VERTEX_POINT ( 'NONE', #1433 ) ;
#83885=DIRECTION ( 'NONE',  ( 0.000000000000000000, 0.000000000000000000, 1.000000000000000000 ) ) ;
#83886=ORIENTED_EDGE ( 'NONE', *, *, #1006, .F. ) ;
#83895=EDGE_LOOP ( 'NONE', ( #55836, #11246, #67602, #32567 ) ) ;
#84022=EDGE_LOOP ( 'NONE', ( #82689, #45786, #36347, #42196 ) ) ;
#84035=VERTEX_POINT ( 'NONE', #36840 ) ;
#84183=PLANE ( 'NONE',  #12 ) ;
#84202=CONICAL_SURFACE ( 'NONE', #76990, 10.66800000000000992, 0.02993239667170383839 ) ;
#84272=VERTEX_POINT ( 'NONE', #73131 ) ;
#84299=VERTEX_POINT ( 'NONE', #40844 ) ;
#84337=ORIENTED_EDGE ( 'NONE', *, *, #16373, .F. ) ;
#84340=FACE_OUTER_BOUND ( 'NONE', #76189, .T. ) ;
#84371=EDGE_CURVE ( 'NONE', #15176, #30425, #10984, .T. ) ;
#84374=DIRECTION ( 'NONE',  ( -1.000000000000000000, 0.000000000000000000, 0.000000000000000000 ) ) ;
#84381=AXIS2_PLACEMENT_3D ( 'NONE', #33047, #18521, #33499 ) ;
#84475=LINE ( 'NONE', #68588, #27607 ) ;
#84488=LINE ( 'NONE', #62667, #11229 ) ;
#84506=ORIENTED_EDGE ( 'NONE', *, *, #65709, .F. ) ;
#84523=LINE ( 'NONE', #21835, #72078 ) ;
#84631=DIRECTION ( 'NONE',  ( 0.000000000000000000, 0.000000000000000000, 1.000000000000000000 ) ) ;
#84665=VERTEX_POINT ( 'NONE', #23574 ) ;
#84677=ADVANCED_FACE ( 'NONE', ( #88474 ), #66664, .T. ) ;
#84683=ADVANCED_FACE ( 'NONE', ( #73479 ), #11253, .F. ) ;
#84769=DIRECTION ( 'NONE',  ( 1.000000000000000000, 0.000000000000000000, 0.000000000000000000 ) ) ;
#84795=EDGE_CURVE ( 'NONE', #78177, #56771, #41189, .T. ) ;
#84810=ORIENTED_EDGE ( 'NONE', *, *, #70012, .T. ) ;
#84828=VERTEX_POINT ( 'NONE', #59672 ) ;
#84843=ORIENTED_EDGE ( 'NONE', *, *, #54541, .T. ) ;
#84846=ORIENTED_EDGE ( 'NONE', *, *, #6795, .T. ) ;
#84868=DIRECTION ( 'NONE',  ( 0.000000000000000000, 0.000000000000000000, 1.000000000000000000 ) ) ;
#84936=EDGE_CURVE ( 'NONE', #64699, #13223, #32871, .T. ) ;
#84978=CARTESIAN_POINT ( 'NONE',  ( 226.4410000000000025, 40.03750000000000142, -2.032000000000000028 ) ) ;
#85008=ORIENTED_EDGE ( 'NONE', *, *, #13000, .F. ) ;
#85056=LINE ( 'NONE', #9187, #38455 ) ;
#85076=ORIENTED_EDGE ( 'NONE', *, *, #303, .T. ) ;
#85085=PRODUCT_DEFINITION_CONTEXT ( 'detailed design', #77131, 'design' ) ;
#85142=DIRECTION ( 'NONE',  ( -1.000000000000000000, 0.000000000000000000, 0.000000000000000000 ) ) ;
#85227=LINE ( 'NONE', #22102, #4572 ) ;
#85233=ORIENTED_EDGE ( 'NONE', *, *, #25587, .T. ) ;
#85266=DIRECTION ( 'NONE',  ( -1.000000000000000000, 0.000000000000000000, -2.108231265501709878E-16 ) ) ;
#85268=AXIS2_PLACEMENT_3D ( 'NONE', #62299, #89576, #20980 ) ;
#85298=EDGE_CURVE ( 'NONE', #42989, #10845, #13322, .T. ) ;
#85300=EDGE_LOOP ( 'NONE', ( #88109, #46409, #80281, #49611 ) ) ;
#85332=VECTOR ( 'NONE', #55432, 1000.000000000000000 ) ;
#85413=SURFACE_STYLE_USAGE ( .BOTH. , #57669 ) ;
#85437=EDGE_CURVE ( 'NONE', #19677, #37178, #18375, .T. ) ;
#85449=DIRECTION ( 'NONE',  ( 0.000000000000000000, 0.000000000000000000, 1.000000000000000000 ) ) ;
#85503=EDGE_CURVE ( 'NONE', #10350, #2727, #30085, .T. ) ;
#85557=ADVANCED_FACE ( 'NONE', ( #17786 ), #19134, .F. ) ;
#85590=CARTESIAN_POINT ( 'NONE',  ( 248.6659999999999968, 52.73749999999999716, -10.97647784993501396 ) ) ;
#85623=ORIENTED_EDGE ( 'NONE', *, *, #49984, .T. ) ;
#85648=CARTESIAN_POINT ( 'NONE',  ( 177.1649999999999920, 14.63749999999999929, -14.28749999999999964 ) ) ;
#85690=CYLINDRICAL_SURFACE ( 'NONE', #51482, 4.762500000000002842 ) ;
#85741=EDGE_CURVE ( 'NONE', #11195, #20936, #479, .T. ) ;
#85742=EDGE_LOOP ( 'NONE', ( #69739, #77698, #70265, #37261 ) ) ;
#85755=LINE ( 'NONE', #77135, #40554 ) ;
#85779=ORIENTED_EDGE ( 'NONE', *, *, #75335, .F. ) ;
#85830=CARTESIAN_POINT ( 'NONE',  ( 204.2160000000000082, 52.73749999999999716, -41.27499999999999858 ) ) ;
#85933=EDGE_CURVE ( 'NONE', #19677, #18647, #84523, .T. ) ;
#85939=FACE_OUTER_BOUND ( 'NONE', #61064, .T. ) ;
#85992=CARTESIAN_POINT ( 'NONE',  ( 248.6659999999999968, 52.73749999999999716, 10.66800000000000104 ) ) ;
#86010=EDGE_CURVE ( 'NONE', #71751, #38623, #24064, .T. ) ;
#86051=CARTESIAN_POINT ( 'NONE',  ( 70.98999999999998067, 52.73749999999999716, -44.45000000000002416 ) ) ;
#86104=DIRECTION ( 'NONE',  ( 0.000000000000000000, 0.000000000000000000, 1.000000000000000000 ) ) ;
#86138=FACE_OUTER_BOUND ( 'NONE', #53165, .T. ) ;
#86177=VERTEX_POINT ( 'NONE', #9984 ) ;
#86211=ORIENTED_EDGE ( 'NONE', *, *, #31867, .F. ) ;
#86225=EDGE_LOOP ( 'NONE', ( #61171, #80751 ) ) ;
#86325=CARTESIAN_POINT ( 'NONE',  ( 205.0097499999990305, 52.73749999999999716, -39.68750000000000000 ) ) ;
#86352=AXIS2_PLACEMENT_3D ( 'NONE', #69682, #76492, #82881 ) ;
#86372=DIRECTION ( 'NONE',  ( 1.000000000000000000, 0.000000000000000000, 0.000000000000000000 ) ) ;
#86387=EDGE_LOOP ( 'NONE', ( #40780, #25308, #36367, #32098 ) ) ;
#86413=DIRECTION ( 'NONE',  ( 1.000000000000000000, 0.000000000000000000, 0.000000000000000000 ) ) ;
#86423=FILL_AREA_STYLE_COLOUR ( '', #59522 ) ;
#86429=DIRECTION ( 'NONE',  ( 1.000000000000000000, -0.000000000000000000, 2.108231265501710124E-16 ) ) ;
#86482=CARTESIAN_POINT ( 'NONE',  ( 257.5940999999999690, 52.73749999999999716, -10.97647784993501396 ) ) ;
#86530=AXIS2_PLACEMENT_3D ( 'NONE', #17314, #23261, #50926 ) ;
#86537=LINE ( 'NONE', #51969, #16361 ) ;
#86549=CYLINDRICAL_SURFACE ( 'NONE', #24264, 8.928099999999993486 ) ;
#86587=EDGE_CURVE ( 'NONE', #83823, #87657, #51632, .T. ) ;
#86619=DIRECTION ( 'NONE',  ( -1.000000000000000000, 0.000000000000000000, 0.000000000000000000 ) ) ;
#86672=VERTEX_POINT ( 'NONE', #16688 ) ;
#86767=ORIENTED_EDGE ( 'NONE', *, *, #6795, .F. ) ;
#86790=DIRECTION ( 'NONE',  ( 1.000000000000000000, 0.000000000000000000, 0.000000000000000000 ) ) ;
#86877=LINE ( 'NONE', #9237, #81336 ) ;
#87031=LINE ( 'NONE', #65240, #38061 ) ;
#87072=DIRECTION ( 'NONE',  ( 0.000000000000000000, 1.000000000000000000, 0.000000000000000000 ) ) ;
#87103=EDGE_LOOP ( 'NONE', ( #52847, #37603, #80006, #44676 ) ) ;
#87105=CIRCLE ( 'NONE', #3007, 3.174999999999997158 ) ;
#87155=PLANE ( 'NONE',  #499 ) ;
#87185=AXIS2_PLACEMENT_3D ( 'NONE', #47808, #6490, #82371 ) ;
#87208=EDGE_CURVE ( 'NONE', #62756, #57314, #34103, .T. ) ;
#87220=CARTESIAN_POINT ( 'NONE',  ( 226.4410000000000025, 65.43750000000000000, 10.66800000000000104 ) ) ;
#87241=EDGE_LOOP ( 'NONE', ( #70236, #38449, #55231, #45990 ) ) ;
#87263=CARTESIAN_POINT ( 'NONE',  ( 248.6659999999999968, 52.73749999999999716, 10.66800000000000104 ) ) ;
#87307=SURFACE_STYLE_FILL_AREA ( #65514 ) ;
#87327=ORIENTED_EDGE ( 'NONE', *, *, #28543, .T. ) ;
#87343=DIRECTION ( 'NONE',  ( 0.000000000000000000, -1.000000000000000000, 0.000000000000000000 ) ) ;
#87372=DIRECTION ( 'NONE',  ( 0.02992792722492364568, 0.000000000000000000, 0.9995520592605569021 ) ) ;
#87421=FACE_BOUND ( 'NONE', #47728, .T. ) ;
#87515=CARTESIAN_POINT ( 'NONE',  ( 177.1649999999999920, 5.112500000000000711, -7.937500000000000000 ) ) ;
#87558=ORIENTED_EDGE ( 'NONE', *, *, #23279, .F. ) ;
#87657=VERTEX_POINT ( 'NONE', #7653 ) ;
#87682=CIRCLE ( 'NONE', #32559, 3.174999999999997158 ) ;
#87702=PLANE ( 'NONE',  #54326 ) ;
#87721=MECHANICAL_DESIGN_GEOMETRIC_PRESENTATION_REPRESENTATION('',(#2145),#52912);
#87722=CARTESIAN_POINT ( 'NONE',  ( 177.1649999999999920, 25.81350000000000477, -7.937500000000000000 ) ) ;
#87741=CARTESIAN_POINT ( 'NONE',  ( 177.1649999999999920, 5.112500000000000711, -58.73749999999999716 ) ) ;
#87755=DIRECTION ( 'NONE',  ( 0.000000000000000000, 0.000000000000000000, -1.000000000000000000 ) ) ;
#87778=CARTESIAN_POINT ( 'NONE',  ( 241.3336515812914911, 65.43750000000000000, 10.66800000000000104 ) ) ;
#87794=CARTESIAN_POINT ( 'NONE',  ( 186.6899999999999977, 52.73749999999999716, -53.97500000000000142 ) ) ;
#87866=CYLINDRICAL_SURFACE ( 'NONE', #42837, 9.524999999999998579 ) ;
#87893=CARTESIAN_POINT ( 'NONE',  ( 238.4043397404674920, 52.73749999999999716, -2.903194600000015502 ) ) ;
#87914=VERTEX_POINT ( 'NONE', #16709 ) ;
#87915=PLANE ( 'NONE',  #32816 ) ;
#88007=ORIENTED_EDGE ( 'NONE', *, *, #36104, .F. ) ;
#88012=FACE_OUTER_BOUND ( 'NONE', #31718, .T. ) ;
#88055=ORIENTED_EDGE ( 'NONE', *, *, #4776, .T. ) ;
#88094=PRODUCT_DEFINITION_SHAPE ( 'NONE', 'NONE',  #32744 ) ;
#88109=ORIENTED_EDGE ( 'NONE', *, *, #14206, .T. ) ;
#88149=FACE_OUTER_BOUND ( 'NONE', #57317, .T. ) ;
#88170=VECTOR ( 'NONE', #10368, 1000.000000000000000 ) ;
#88364=EDGE_LOOP ( 'NONE', ( #74812, #31565, #76007, #4515 ) ) ;
#88384=VERTEX_POINT ( 'NONE', #17923 ) ;
#88466=AXIS2_PLACEMENT_3D ( 'NONE', #86051, #51490, #16552 ) ;
#88474=FACE_OUTER_BOUND ( 'NONE', #61009, .T. ) ;
#88508=ORIENTED_EDGE ( 'NONE', *, *, #12325, .T. ) ;
#88584=ORIENTED_EDGE ( 'NONE', *, *, #52777, .F. ) ;
#88609=CARTESIAN_POINT ( 'NONE',  ( 223.2659999999999911, 52.73749999999999716, -44.45000000000000284 ) ) ;
#88646=CARTESIAN_POINT ( 'NONE',  ( 255.9983484187079910, 40.03750000000000142, -2.032000000000000028 ) ) ;
#88663=CARTESIAN_POINT ( 'NONE',  ( 270.8910000000000196, 40.03750000000000142, -58.73749999999999716 ) ) ;
#88678=CARTESIAN_POINT ( 'NONE',  ( 245.4909999999999854, 65.43750000000000000, -67.11950000000000216 ) ) ;
#88690=LINE ( 'NONE', #47313, #55048 ) ;
#88778=DIRECTION ( 'NONE',  ( 1.000000000000000000, 0.000000000000000000, 0.000000000000000000 ) ) ;
#88784=CARTESIAN_POINT ( 'NONE',  ( 237.9979999999999905, 52.73749999999999716, 10.66800000000000104 ) ) ;
#88844=EDGE_LOOP ( 'NONE', ( #69051, #54970 ) ) ;
#89035=ORIENTED_EDGE ( 'NONE', *, *, #49065, .T. ) ;
#89046=DIRECTION ( 'NONE',  ( 1.000000000000000000, 0.000000000000000000, 0.000000000000000000 ) ) ;
#89051=LINE ( 'NONE', #73626, #41009 ) ;
#89116=DIRECTION ( 'NONE',  ( 1.000000000000000000, 0.000000000000000000, 0.000000000000000000 ) ) ;
#89122=CARTESIAN_POINT ( 'NONE',  ( 270.8910000000000196, 65.43750000000000000, -67.11950000000000216 ) ) ;
#89174=FACE_OUTER_BOUND ( 'NONE', #16683, .T. ) ;
#89214=CARTESIAN_POINT ( 'NONE',  ( 199.3900000000000148, 52.73749999999999716, -47.62500000000000000 ) ) ;
#89249=ORIENTED_EDGE ( 'NONE', *, *, #55904, .T. ) ;
#89339=EDGE_CURVE ( 'NONE', #73485, #78558, #40669, .T. ) ;
#89416=VERTEX_POINT ( 'NONE', #30001 ) ;
#89458=VECTOR ( 'NONE', #3711, 1000.000000000000000 ) ;
#89484=ORIENTED_EDGE ( 'NONE', *, *, #82703, .F. ) ;
#89547=VECTOR ( 'NONE', #54770, 1000.000000000000000 ) ;
#89576=DIRECTION ( 'NONE',  ( 0.7071067811865480168, -0.7071067811865470176, 0.000000000000000000 ) ) ;
#89596=DIRECTION ( 'NONE',  ( 0.000000000000000000, 0.000000000000000000, -1.000000000000000000 ) ) ;
#89656=CARTESIAN_POINT ( 'NONE',  ( 0.000000000000000000, 0.000000000000000000, 0.000000000000000000 ) ) ;
#89718=ORIENTED_EDGE ( 'NONE', *, *, #8349, .F. ) ;
#89736=DIRECTION ( 'NONE',  ( 0.000000000000000000, 0.000000000000000000, 1.000000000000000000 ) ) ;
ENDSEC;
END-ISO-10303-21;
